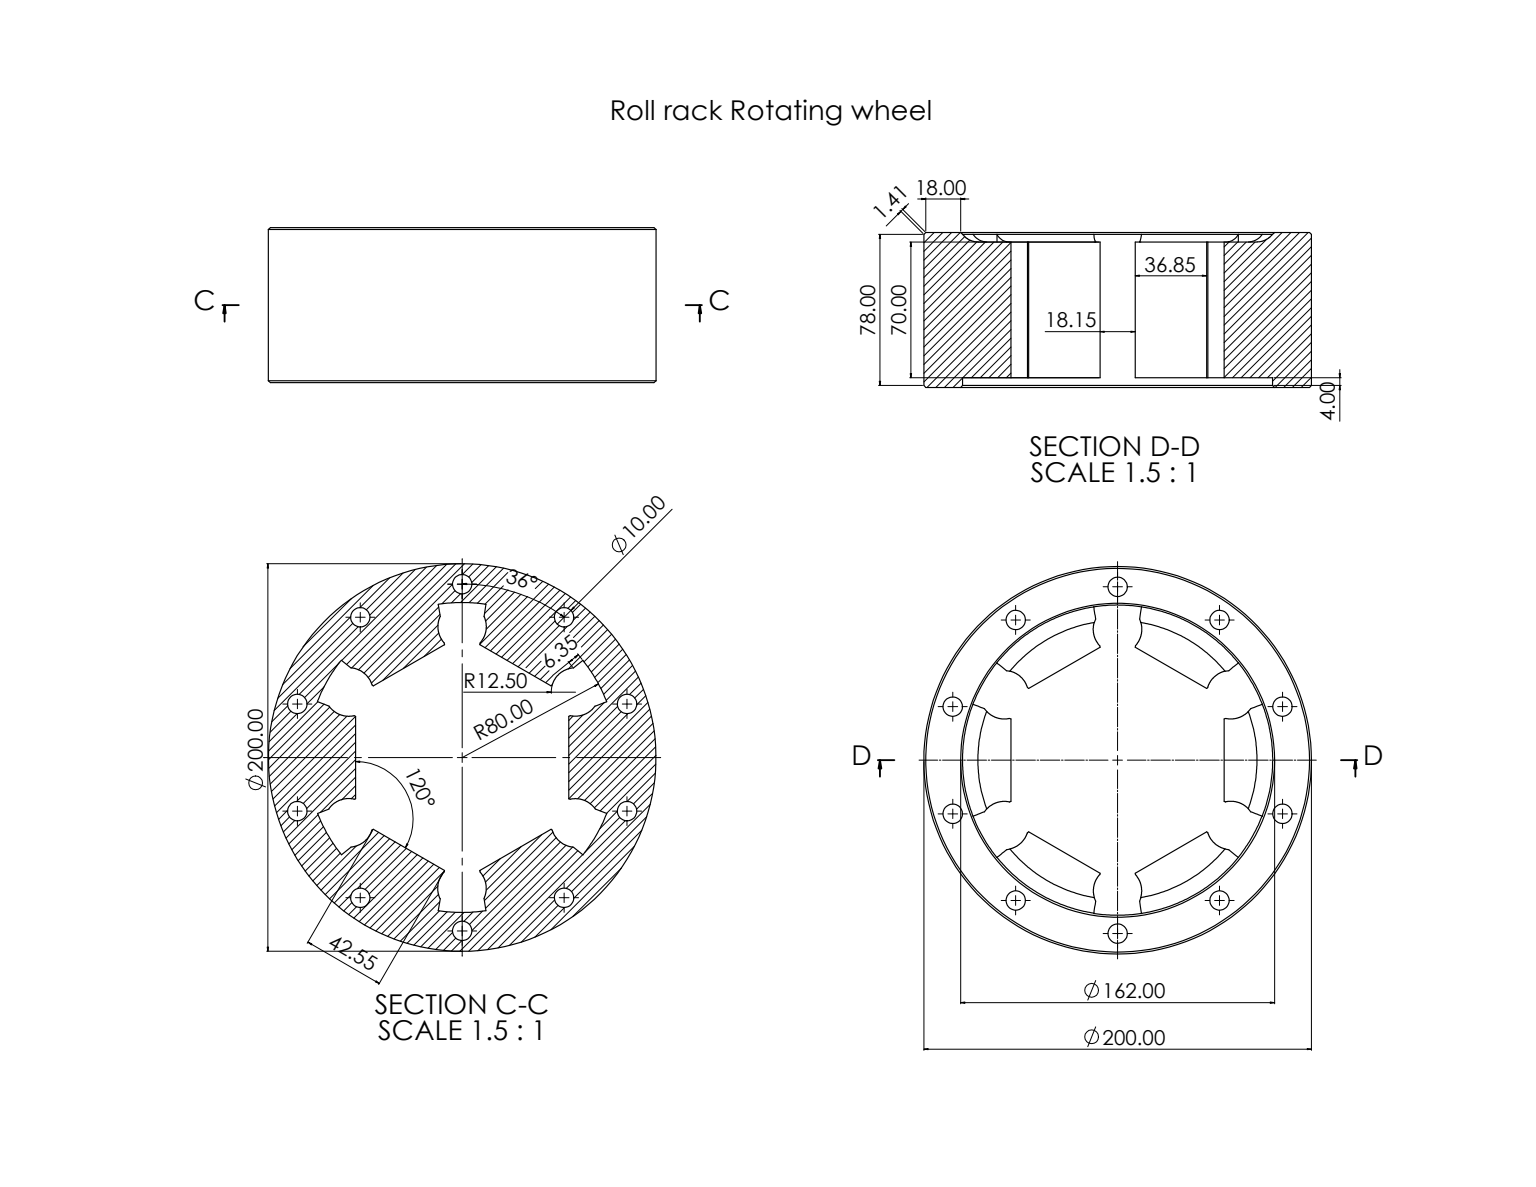
ISO-10303-21;
HEADER;
FILE_DESCRIPTION (('STEP AP214'),
    '1' );
FILE_NAME ('Roll rack Rotating wheel.step',
    '2026-10-25T19:19:31',
    ( '' ),
    ( '' ),
    'SwSTEP 2.0',
    'SolidWorks 2025',
    '' );
FILE_SCHEMA (( 'AUTOMOTIVE_DESIGN' ));
ENDSEC;

DATA;
#2=AXIS2_PLACEMENT_3D ( 'NONE', #924, #2806, #4329 ) ;
#5=ORIENTED_EDGE ( 'NONE', *, *, #469, .T. ) ;
#9=EDGE_CURVE ( 'NONE', #3175, #2261, #1933, .T. ) ;
#11=EDGE_LOOP ( 'NONE', ( #620, #96, #4571, #312 ) ) ;
#12=DIRECTION ( 'NONE',  ( 0.6273063437270283149, 0.7787725926866119197, -0.000000000000000000 ) ) ;
#15=VERTEX_POINT ( 'NONE', #3832 ) ;
#16=ORIENTED_EDGE ( 'NONE', *, *, #1748, .F. ) ;
#17=LINE ( 'NONE', #2869, #5066 ) ;
#21=EDGE_CURVE ( 'NONE', #4952, #1308, #564, .T. ) ;
#24=ORIENTED_EDGE ( 'NONE', *, *, #3439, .T. ) ;
#27=FACE_OUTER_BOUND ( 'NONE', #743, .T. ) ;
#28=ORIENTED_EDGE ( 'NONE', *, *, #3600, .T. ) ;
#29=CARTESIAN_POINT ( 'NONE',  ( -27.50000000000000355, -47.63139720814412215, 35.00000000000000000 ) ) ;
#30=CARTESIAN_POINT ( 'NONE',  ( 0.000000000000000000, -67.50000000000000000, 35.00000000000000000 ) ) ;
#32=CARTESIAN_POINT ( 'NONE',  ( -68.69027832784050247, 26.57196568621489163, 35.13717928826310555 ) ) ;
#33=ORIENTED_EDGE ( 'NONE', *, *, #1361, .F. ) ;
#34=CARTESIAN_POINT ( 'NONE',  ( 0.000000000000000000, 0.000000000000000000, -39.00000000000002842 ) ) ;
#36=DIRECTION ( 'NONE',  ( -0.000000000000000000, -0.000000000000000000, -1.000000000000000000 ) ) ;
#37=VERTEX_POINT ( 'NONE', #2442 ) ;
#42=ORIENTED_EDGE ( 'NONE', *, *, #5266, .F. ) ;
#43=ORIENTED_EDGE ( 'NONE', *, *, #3427, .F. ) ;
#44=DIRECTION ( 'NONE',  ( 1.000000000000000000, 0.000000000000000000, 0.000000000000000000 ) ) ;
#45=LINE ( 'NONE', #2928, #381 ) ;
#48=EDGE_CURVE ( 'NONE', #2705, #6084, #5252, .T. ) ;
#52=CARTESIAN_POINT ( 'NONE',  ( -85.08403291566554572, 27.64547812922971914, -40.00000000000000000 ) ) ;
#53=AXIS2_PLACEMENT_3D ( 'NONE', #2121, #1570, #3471 ) ;
#55=DIRECTION ( 'NONE',  ( -0.000000000000000000, -0.000000000000000000, -1.000000000000000000 ) ) ;
#58=AXIS2_PLACEMENT_3D ( 'NONE', #3243, #1826, #3726 ) ;
#65=AXIS2_PLACEMENT_3D ( 'NONE', #52, #3436, #1534 ) ;
#67=LINE ( 'NONE', #4284, #175 ) ;
#68=AXIS2_PLACEMENT_3D ( 'NONE', #5525, #4167, #5643 ) ;
#70=LINE ( 'NONE', #4287, #2332 ) ;
#71=ORIENTED_EDGE ( 'NONE', *, *, #3542, .T. ) ;
#72=LINE ( 'NONE', #3851, #3967 ) ;
#73=AXIS2_PLACEMENT_3D ( 'NONE', #3304, #3763, #5645 ) ;
#76=ORIENTED_EDGE ( 'NONE', *, *, #3903, .F. ) ;
#78=ORIENTED_EDGE ( 'NONE', *, *, #3494, .T. ) ;
#79=DIRECTION ( 'NONE',  ( -0.000000000000000000, -0.000000000000000000, 1.000000000000000000 ) ) ;
#84=CARTESIAN_POINT ( 'NONE',  ( 58.45671475545002949, -33.74999999999933209, 35.00000000000000000 ) ) ;
#86=VECTOR ( 'NONE', #3244, 1000.000000000000114 ) ;
#88=CARTESIAN_POINT ( 'NONE',  ( -4.130675435985315210E-14, -1.067806758184287486E-13, -35.00000000000000000 ) ) ;
#89=DIRECTION ( 'NONE',  ( -0.000000000000000000, -0.000000000000000000, 1.000000000000000000 ) ) ;
#91=ORIENTED_EDGE ( 'NONE', *, *, #553, .T. ) ;
#92=CYLINDRICAL_SURFACE ( 'NONE', #5438, 12.50000000000000355 ) ;
#93=CIRCLE ( 'NONE', #494, 100.0000000000000000 ) ;
#95=VECTOR ( 'NONE', #4136, 1000.000000000000000 ) ;
#96=ORIENTED_EDGE ( 'NONE', *, *, #2491, .F. ) ;
#97=VECTOR ( 'NONE', #2993, 1000.000000000000000 ) ;
#99=EDGE_CURVE ( 'NONE', #3250, #2370, #287, .T. ) ;
#103=VERTEX_POINT ( 'NONE', #3026 ) ;
#104=DIRECTION ( 'NONE',  ( 1.000000000000000000, 0.000000000000000000, 0.000000000000000000 ) ) ;
#106=CARTESIAN_POINT ( 'NONE',  ( 90.08403291566575888, -27.64547812922912939, -40.00000000000000000 ) ) ;
#107=ORIENTED_EDGE ( 'NONE', *, *, #3615, .T. ) ;
#110=ORIENTED_EDGE ( 'NONE', *, *, #2448, .F. ) ;
#111=ORIENTED_EDGE ( 'NONE', *, *, #3009, .T. ) ;
#112=DIRECTION ( 'NONE',  ( -1.000000000000000000, 0.000000000000000000, 0.000000000000000000 ) ) ;
#117=ORIENTED_EDGE ( 'NONE', *, *, #561, .F. ) ;
#123=ORIENTED_EDGE ( 'NONE', *, *, #596, .F. ) ;
#126=ORIENTED_EDGE ( 'NONE', *, *, #1149, .F. ) ;
#128=EDGE_CURVE ( 'NONE', #3596, #4984, #485, .T. ) ;
#130=EDGE_CURVE ( 'NONE', #3466, #5138, #2058, .T. ) ;
#132=VERTEX_POINT ( 'NONE', #187 ) ;
#135=CARTESIAN_POINT ( 'NONE',  ( 11.82353433160363387, 71.60642589802917257, 35.00000000000000000 ) ) ;
#138=EDGE_CURVE ( 'NONE', #2272, #193, #3964, .T. ) ;
#139=ORIENTED_EDGE ( 'NONE', *, *, #5184, .F. ) ;
#140=ORIENTED_EDGE ( 'NONE', *, *, #2807, .F. ) ;
#142=DIRECTION ( 'NONE',  ( -0.4999999999999919509, -0.8660254037844432595, 0.000000000000000000 ) ) ;
#143=DIRECTION ( 'NONE',  ( 0.8660254037844374864, 0.5000000000000018874, 0.000000000000000000 ) ) ;
#144=CARTESIAN_POINT ( 'NONE',  ( 55.71784976887228424, -21.55374571496028224, -35.00000000000000000 ) ) ;
#148=CARTESIAN_POINT ( 'NONE',  ( -99.00000000000005684, 0.000000000000000000, 40.00000000000000000 ) ) ;
#152=ORIENTED_EDGE ( 'NONE', *, *, #4059, .F. ) ;
#154=EDGE_CURVE ( 'NONE', #2132, #2202, #3672, .T. ) ;
#155=CIRCLE ( 'NONE', #3811, 12.50000000000138733 ) ;
#157=CARTESIAN_POINT ( 'NONE',  ( -67.92475106770436355, 25.56373185532726566, 35.00000000000000000 ) ) ;
#158=ORIENTED_EDGE ( 'NONE', *, *, #5715, .F. ) ;
#159=FACE_OUTER_BOUND ( 'NONE', #3787, .T. ) ;
#160=CIRCLE ( 'NONE', #3618, 5.000000000000004441 ) ;
#162=CIRCLE ( 'NONE', #672, 99.00000000000005684 ) ;
#163=LINE ( 'NONE', #3014, #5926 ) ;
#165=AXIS2_PLACEMENT_3D ( 'NONE', #2293, #4791, #5233 ) ;
#166=CARTESIAN_POINT ( 'NONE',  ( -90.08403291566554572, 27.64547812922971914, 40.00000000000000000 ) ) ;
#170=AXIS2_PLACEMENT_3D ( 'NONE', #2221, #6035, #3192 ) ;
#171=ORIENTED_EDGE ( 'NONE', *, *, #1511, .T. ) ;
#173=ORIENTED_EDGE ( 'NONE', *, *, #319, .F. ) ;
#174=PLANE ( 'NONE',  #2670 ) ;
#175=VECTOR ( 'NONE', #443, 1000.000000000000000 ) ;
#177=DIRECTION ( 'NONE',  ( 0.000000000000000000, 0.000000000000000000, 1.000000000000000000 ) ) ;
#179=AXIS2_PLACEMENT_3D ( 'NONE', #1316, #5314, #565 ) ;
#182=DIRECTION ( 'NONE',  ( -0.000000000000000000, -0.000000000000000000, -1.000000000000000000 ) ) ;
#183=ORIENTED_EDGE ( 'NONE', *, *, #3874, .T. ) ;
#184=VECTOR ( 'NONE', #2953, 1000.000000000000000 ) ;
#187=CARTESIAN_POINT ( 'NONE',  ( -11.33314185116896589, -72.77350886803867525, -35.00000000000000000 ) ) ;
#188=FACE_OUTER_BOUND ( 'NONE', #757, .T. ) ;
#189=AXIS2_PLACEMENT_3D ( 'NONE', #1496, #4390, #4322 ) ;
#190=ORIENTED_EDGE ( 'NONE', *, *, #4573, .T. ) ;
#191=DIRECTION ( 'NONE',  ( -1.000000000000000000, 0.000000000000000000, 0.000000000000000000 ) ) ;
#193=VERTEX_POINT ( 'NONE', #6023 ) ;
#197=AXIS2_PLACEMENT_3D ( 'NONE', #5583, #3182, #1309 ) ;
#199=EDGE_LOOP ( 'NONE', ( #4634, #1674, #4035, #780 ) ) ;
#200=CARTESIAN_POINT ( 'NONE',  ( -56.72666074499610289, 46.14586675604117971, 35.04915833130703362 ) ) ;
#201=CIRCLE ( 'NONE', #4460, 80.99999999999998579 ) ;
#204=ORIENTED_EDGE ( 'NONE', *, *, #2780, .T. ) ;
#206=ORIENTED_EDGE ( 'NONE', *, *, #6021, .F. ) ;
#208=EDGE_CURVE ( 'NONE', #3788, #4471, #2464, .T. ) ;
#209=ADVANCED_FACE ( 'NONE', ( #3211 ), #1827, .F. ) ;
#210=CARTESIAN_POINT ( 'NONE',  ( 85.08403291566575888, -27.64547812922912939, -79.99999999999998579 ) ) ;
#212=VECTOR ( 'NONE', #3452, 1000.000000000000000 ) ;
#213=LINE ( 'NONE', #3513, #2487 ) ;
#214=DIRECTION ( 'NONE',  ( -0.1538769332794359124, -0.9880900209011910240, 0.000000000000000000 ) ) ;
#216=ORIENTED_EDGE ( 'NONE', *, *, #469, .F. ) ;
#218=CARTESIAN_POINT ( 'NONE',  ( 85.08403291566575888, -27.64547812922912939, -79.99999999999998579 ) ) ;
#220=CARTESIAN_POINT ( 'NONE',  ( 58.45671475545002949, -33.74999999999933209, -35.00000000000000000 ) ) ;
#221=ORIENTED_EDGE ( 'NONE', *, *, #961, .T. ) ;
#222=CARTESIAN_POINT ( 'NONE',  ( 0.000000000000000000, 67.50000000000000000, 35.00000000000000000 ) ) ;
#227=PLANE ( 'NONE',  #262 ) ;
#228=EDGE_LOOP ( 'NONE', ( #2833, #2613, #5, #4505, #3148 ) ) ;
#229=DIRECTION ( 'NONE',  ( -0.000000000000000000, -0.000000000000000000, 1.000000000000000000 ) ) ;
#230=DIRECTION ( 'NONE',  ( 1.000000000000000000, 0.000000000000000000, 0.000000000000000000 ) ) ;
#234=ORIENTED_EDGE ( 'NONE', *, *, #392, .F. ) ;
#236=LINE ( 'NONE', #1613, #5345 ) ;
#238=CARTESIAN_POINT ( 'NONE',  ( 0.000000000000000000, 0.000000000000000000, 45.00000000000000711 ) ) ;
#239=CARTESIAN_POINT ( 'NONE',  ( -52.58482424179536707, 72.37680137756343868, 40.00000000000000000 ) ) ;
#241=EDGE_CURVE ( 'NONE', #1987, #2346, #2214, .T. ) ;
#245=PLANE ( 'NONE',  #776 ) ;
#246=ORIENTED_EDGE ( 'NONE', *, *, #2518, .T. ) ;
#247=PLANE ( 'NONE',  #2430 ) ;
#252=DIRECTION ( 'NONE',  ( -0.000000000000000000, -0.000000000000000000, -1.000000000000000000 ) ) ;
#256=ORIENTED_EDGE ( 'NONE', *, *, #1736, .F. ) ;
#257=ORIENTED_EDGE ( 'NONE', *, *, #4805, .F. ) ;
#258=VECTOR ( 'NONE', #4022, 1000.000000000000000 ) ;
#261=LINE ( 'NONE', #1193, #1745 ) ;
#262=AXIS2_PLACEMENT_3D ( 'NONE', #791, #5542, #322 ) ;
#264=CARTESIAN_POINT ( 'NONE',  ( -55.00000000000000711, -2.463307335887066074E-13, -35.00000000000000000 ) ) ;
#267=FACE_OUTER_BOUND ( 'NONE', #1954, .T. ) ;
#268=CARTESIAN_POINT ( 'NONE',  ( 58.45671475545002949, -33.74999999999933209, 35.00000000000000000 ) ) ;
#269=AXIS2_PLACEMENT_3D ( 'NONE', #1659, #727, #3101 ) ;
#270=AXIS2_PLACEMENT_3D ( 'NONE', #5191, #932, #5592 ) ;
#275=CARTESIAN_POINT ( 'NONE',  ( -57.35713647666923976, 46.20154318182412112, -35.00000000000000000 ) ) ;
#276=AXIS2_PLACEMENT_3D ( 'NONE', #3833, #3374, #536 ) ;
#277=AXIS2_PLACEMENT_3D ( 'NONE', #5004, #3496, #662 ) ;
#279=CARTESIAN_POINT ( 'NONE',  ( -99.00000000000000000, 1.218523565151616460E-14, -40.00000000000000000 ) ) ;
#282=ORIENTED_EDGE ( 'NONE', *, *, #3578, .T. ) ;
#283=AXIS2_PLACEMENT_3D ( 'NONE', #2617, #2590, #2677 ) ;
#284=PLANE ( 'NONE',  #4114 ) ;
#286=FACE_OUTER_BOUND ( 'NONE', #5823, .T. ) ;
#287=CIRCLE ( 'NONE', #788, 80.00000000000000000 ) ;
#288=FACE_OUTER_BOUND ( 'NONE', #4896, .T. ) ;
#290=ORIENTED_EDGE ( 'NONE', *, *, #3576, .F. ) ;
#291=ORIENTED_EDGE ( 'NONE', *, *, #9, .T. ) ;
#295=ORIENTED_EDGE ( 'NONE', *, *, #6012, .F. ) ;
#299=PLANE ( 'NONE',  #2579 ) ;
#300=CARTESIAN_POINT ( 'NONE',  ( 57.35713647667095927, 46.20154318182582642, 35.00000000000000000 ) ) ;
#302=AXIS2_PLACEMENT_3D ( 'NONE', #2834, #4360, #112 ) ;
#309=CIRCLE ( 'NONE', #2876, 12.49999999999999822 ) ;
#311=DIRECTION ( 'NONE',  ( -0.7787725926866080339, -0.6273063437270329779, 0.000000000000000000 ) ) ;
#312=ORIENTED_EDGE ( 'NONE', *, *, #2008, .T. ) ;
#313=PRODUCT_DEFINITION ( 'UNKNOWN', '', #4945, #1510 ) ;
#316=ORIENTED_EDGE ( 'NONE', *, *, #3343, .F. ) ;
#319=EDGE_CURVE ( 'NONE', #3286, #747, #5307, .T. ) ;
#322=DIRECTION ( 'NONE',  ( -0.9326495259660518844, 0.3607836771741465554, 0.000000000000000000 ) ) ;
#324=EDGE_CURVE ( 'NONE', #559, #1473, #4803, .T. ) ;
#326=ORIENTED_EDGE ( 'NONE', *, *, #3380, .T. ) ;
#332=LINE ( 'NONE', #833, #5327 ) ;
#334=EDGE_CURVE ( 'NONE', #2774, #836, #5704, .T. ) ;
#335=CARTESIAN_POINT ( 'NONE',  ( -45.92560378283280187, -36.99336990414421678, 35.00000000000000000 ) ) ;
#337=CARTESIAN_POINT ( 'NONE',  ( -80.00000000000000000, 9.858406733136196781E-15, 38.99999999999995737 ) ) ;
#339=DIRECTION ( 'NONE',  ( 0.8660254037844374864, 0.5000000000000018874, 0.000000000000000000 ) ) ;
#345=DIRECTION ( 'NONE',  ( 0.4999999999999979461, 0.8660254037844397068, 0.000000000000000000 ) ) ;
#346=CARTESIAN_POINT ( 'NONE',  ( 0.000000000000000000, 0.000000000000000000, -35.00000000000000000 ) ) ;
#347=CARTESIAN_POINT ( 'NONE',  ( 80.00000000000000000, 9.797174393178826052E-15, -35.00000000000000000 ) ) ;
#348=DIRECTION ( 'NONE',  ( 0.9326495259660493309, -0.3607836771741531612, 0.000000000000000000 ) ) ;
#352=ORIENTED_EDGE ( 'NONE', *, *, #5211, .T. ) ;
#355=LINE ( 'NONE', #765, #5264 ) ;
#356=LINE ( 'NONE', #854, #4752 ) ;
#357=ADVANCED_FACE ( 'NONE', ( #528 ), #1432, .F. ) ;
#358=CYLINDRICAL_SURFACE ( 'NONE', #2932, 5.000000000000005329 ) ;
#361=CIRCLE ( 'NONE', #2438, 5.000000000000003553 ) ;
#362=EDGE_LOOP ( 'NONE', ( #5160, #1425, #4288, #5479, #680 ) ) ;
#364=CYLINDRICAL_SURFACE ( 'NONE', #2030, 5.000000000000004441 ) ;
#366=EDGE_CURVE ( 'NONE', #3309, #2604, #45, .T. ) ;
#367=VECTOR ( 'NONE', #4179, 1000.000000000000000 ) ;
#371=AXIS2_PLACEMENT_3D ( 'NONE', #5124, #1347, #5615 ) ;
#372=ORIENTED_EDGE ( 'NONE', *, *, #1885, .T. ) ;
#373=AXIS2_PLACEMENT_3D ( 'NONE', #5753, #1444, #5257 ) ;
#375=DIRECTION ( 'NONE',  ( 0.1538769332794487910, -0.9880900209011889146, 0.000000000000000000 ) ) ;
#378=DIRECTION ( 'NONE',  ( 0.9880900209011890256, 0.1538769332794488465, -0.000000000000000000 ) ) ;
#379=CARTESIAN_POINT ( 'NONE',  ( -1.131281550719566266E-13, -1.761763928569765259E-14, -35.00000000000000000 ) ) ;
#381=VECTOR ( 'NONE', #2434, 1000.000000000000000 ) ;
#385=DIRECTION ( 'NONE',  ( 0.4999999999999980016, 0.8660254037844398178, 0.000000000000000000 ) ) ;
#386=DIRECTION ( 'NONE',  ( 0.7071067811865474617, 8.659560562354932858E-17, -0.7071067811865474617 ) ) ;
#387=CARTESIAN_POINT ( 'NONE',  ( 0.000000000000000000, 0.000000000000000000, -35.00000000000000000 ) ) ;
#389=CIRCLE ( 'NONE', #3743, 81.00000000000004263 ) ;
#390=CARTESIAN_POINT ( 'NONE',  ( -46.52501622030417394, 37.47620048660903080, -35.00000000000000000 ) ) ;
#391=ADVANCED_FACE ( 'NONE', ( #4837 ), #4296, .F. ) ;
#392=EDGE_CURVE ( 'NONE', #6119, #506, #4546, .T. ) ;
#393=CIRCLE ( 'NONE', #4250, 5.000000000000004441 ) ;
#394=ORIENTED_EDGE ( 'NONE', *, *, #319, .T. ) ;
#395=FACE_OUTER_BOUND ( 'NONE', #5732, .T. ) ;
#396=CARTESIAN_POINT ( 'NONE',  ( 45.92560378283280187, 36.99336990414421678, 35.00000000000000000 ) ) ;
#398=AXIS2_PLACEMENT_3D ( 'NONE', #2597, #2507, #3090 ) ;
#403=VECTOR ( 'NONE', #3278, 1000.000000000000000 ) ;
#404=VERTEX_POINT ( 'NONE', #2337 ) ;
#406=CARTESIAN_POINT ( 'NONE',  ( 57.35713647666955950, -46.20154318182373032, 35.13717928826270054 ) ) ;
#407=ORIENTED_EDGE ( 'NONE', *, *, #3155, .F. ) ;
#408=CARTESIAN_POINT ( 'NONE',  ( -47.58482424179695158, -72.37680137756228760, -79.99999999999998579 ) ) ;
#409=EDGE_CURVE ( 'NONE', #4283, #4835, #4739, .T. ) ;
#410=CARTESIAN_POINT ( 'NONE',  ( 45.92560378283317135, -36.99336990414376913, -35.00000000000000000 ) ) ;
#411=LINE ( 'NONE', #2288, #367 ) ;
#413=VERTEX_POINT ( 'NONE', #3086 ) ;
#415=EDGE_LOOP ( 'NONE', ( #3992, #873, #2536, #5412 ) ) ;
#417=CARTESIAN_POINT ( 'NONE',  ( -54.99999999999990052, -21.27605460800010206, 35.00000000000000000 ) ) ;
#418=CARTESIAN_POINT ( 'NONE',  ( 0.000000000000000000, 0.000000000000000000, 38.99999999999995737 ) ) ;
#419=ORIENTED_EDGE ( 'NONE', *, *, #6088, .T. ) ;
#421=DIRECTION ( 'NONE',  ( 0.000000000000000000, 0.000000000000000000, 1.000000000000000000 ) ) ;
#422=ORIENTED_EDGE ( 'NONE', *, *, #959, .T. ) ;
#424=DIRECTION ( 'NONE',  ( -0.000000000000000000, -0.000000000000000000, -1.000000000000000000 ) ) ;
#426=ADVANCED_FACE ( 'NONE', ( #4483 ), #2145, .F. ) ;
#428=CARTESIAN_POINT ( 'NONE',  ( 0.000000000000000000, -67.50000000000000000, 35.00000000000000000 ) ) ;
#429=VERTEX_POINT ( 'NONE', #3953 ) ;
#431=LINE ( 'NONE', #905, #1941 ) ;
#432=EDGE_CURVE ( 'NONE', #3051, #2891, #3112, .T. ) ;
#433=ADVANCED_FACE ( 'NONE', ( #2109 ), #652, .T. ) ;
#434=ORIENTED_EDGE ( 'NONE', *, *, #2926, .T. ) ;
#435=DIRECTION ( 'NONE',  ( 0.4999999999999980571, 0.8660254037844398178, 0.000000000000000000 ) ) ;
#438=EDGE_CURVE ( 'NONE', #2727, #2151, #236, .T. ) ;
#439=CARTESIAN_POINT ( 'NONE',  ( 0.000000000000000000, 0.000000000000000000, 40.00000000000000000 ) ) ;
#441=CARTESIAN_POINT ( 'NONE',  ( -9.192833548570002122, 59.02994620156853500, 35.00000000000000000 ) ) ;
#442=ORIENTED_EDGE ( 'NONE', *, *, #4598, .F. ) ;
#443=DIRECTION ( 'NONE',  ( -0.000000000000000000, -0.000000000000000000, -1.000000000000000000 ) ) ;
#446=ORIENTED_EDGE ( 'NONE', *, *, #3414, .T. ) ;
#447=DIRECTION ( 'NONE',  ( -0.9326495259660493309, 0.3607836771741531612, 0.000000000000000000 ) ) ;
#448=CARTESIAN_POINT ( 'NONE',  ( 0.000000000000000000, 0.000000000000000000, 39.00000000000007105 ) ) ;
#449=ORIENTED_EDGE ( 'NONE', *, *, #4908, .F. ) ;
#454=CARTESIAN_POINT ( 'NONE',  ( 67.15076586955507310, 25.97642475654038208, 45.00000000000000711 ) ) ;
#455=DIRECTION ( 'NONE',  ( -0.000000000000000000, -0.000000000000000000, -1.000000000000000000 ) ) ;
#456=VECTOR ( 'NONE', #3870, 1000.000000000000000 ) ;
#457=ORIENTED_EDGE ( 'NONE', *, *, #2284, .T. ) ;
#460=ORIENTED_EDGE ( 'NONE', *, *, #2064, .F. ) ;
#461=DIRECTION ( 'NONE',  ( -0.1538769332794359124, -0.9880900209011910240, 0.000000000000000000 ) ) ;
#462=CIRCLE ( 'NONE', #5923, 10.00000000000000000 ) ;
#463=CIRCLE ( 'NONE', #5827, 80.00000000000000000 ) ;
#465=CARTESIAN_POINT ( 'NONE',  ( 0.000000000000000000, 0.000000000000000000, 40.00000000000000000 ) ) ;
#469=EDGE_CURVE ( 'NONE', #4283, #4976, #5856, .T. ) ;
#470=CARTESIAN_POINT ( 'NONE',  ( 57.35713647667095927, 46.20154318182582642, -35.00000000000000000 ) ) ;
#471=AXIS2_PLACEMENT_3D ( 'NONE', #3650, #3190, #2720 ) ;
#472=CIRCLE ( 'NONE', #5133, 5.000000000000004441 ) ;
#474=CARTESIAN_POINT ( 'NONE',  ( 46.52501622030217021, 37.47620048660763103, 35.00000000000000000 ) ) ;
#477=ORIENTED_EDGE ( 'NONE', *, *, #4239, .T. ) ;
#478=DIRECTION ( 'NONE',  ( 0.000000000000000000, 0.000000000000000000, 1.000000000000000000 ) ) ;
#480=CIRCLE ( 'NONE', #3045, 5.000000000000004441 ) ;
#481=LINE ( 'NONE', #2362, #700 ) ;
#482=CYLINDRICAL_SURFACE ( 'NONE', #4115, 12.49999999999999822 ) ;
#483=ORIENTED_EDGE ( 'NONE', *, *, #1361, .T. ) ;
#484=LINE ( 'NONE', #4827, #2071 ) ;
#485=CIRCLE ( 'NONE', #982, 12.50000000000138556 ) ;
#491=DIRECTION ( 'NONE',  ( 0.7787725926866119197, -0.6273063437270283149, 0.000000000000000000 ) ) ;
#492=CARTESIAN_POINT ( 'NONE',  ( -55.71784976887420271, -21.55374571496209057, 35.00000000000000000 ) ) ;
#494=AXIS2_PLACEMENT_3D ( 'NONE', #1360, #5019, #5052 ) ;
#496=DIRECTION ( 'NONE',  ( -0.000000000000000000, -0.000000000000000000, 1.000000000000000000 ) ) ;
#501=AXIS2_PLACEMENT_3D ( 'NONE', #5606, #4101, #6017 ) ;
#503=DIRECTION ( 'NONE',  ( 4.496403249731883200E-15, -1.000000000000000000, 0.000000000000000000 ) ) ;
#504=EDGE_CURVE ( 'NONE', #1915, #1987, #3073, .T. ) ;
#505=CIRCLE ( 'NONE', #3166, 10.00000000000000178 ) ;
#506=VERTEX_POINT ( 'NONE', #1560 ) ;
#507=DIRECTION ( 'NONE',  ( -0.000000000000000000, -0.000000000000000000, -1.000000000000000000 ) ) ;
#508=CIRCLE ( 'NONE', #5964, 12.50000000000000355 ) ;
#510=CYLINDRICAL_SURFACE ( 'NONE', #4830, 12.49999999999999822 ) ;
#511=AXIS2_PLACEMENT_3D ( 'NONE', #4477, #2587, #1635 ) ;
#512=ADVANCED_FACE ( 'NONE', ( #3981 ), #3487, .F. ) ;
#517=DIRECTION ( 'NONE',  ( 0.5000000000000099920, -0.8660254037844329345, 0.000000000000000000 ) ) ;
#518=LINE ( 'NONE', #4350, #5754 ) ;
#519=FACE_OUTER_BOUND ( 'NONE', #1704, .T. ) ;
#524=ORIENTED_EDGE ( 'NONE', *, *, #5142, .T. ) ;
#528=FACE_OUTER_BOUND ( 'NONE', #1887, .T. ) ;
#530=DIRECTION ( 'NONE',  ( 0.3607836771741718129, -0.9326495259660421144, 0.000000000000000000 ) ) ;
#531=EDGE_CURVE ( 'NONE', #5256, #4984, #2504, .T. ) ;
#536=DIRECTION ( 'NONE',  ( 1.000000000000000000, 0.000000000000000000, 0.000000000000000000 ) ) ;
#537=VERTEX_POINT ( 'NONE', #4039 ) ;
#538=LINE ( 'NONE', #2882, #759 ) ;
#543=ORIENTED_EDGE ( 'NONE', *, *, #2903, .T. ) ;
#545=CARTESIAN_POINT ( 'NONE',  ( -57.58482424179695869, -72.37680137756228760, 40.00000000000000000 ) ) ;
#549=ORIENTED_EDGE ( 'NONE', *, *, #553, .F. ) ;
#552=DIRECTION ( 'NONE',  ( 1.000000000000000000, 0.000000000000000000, 0.000000000000000000 ) ) ;
#553=EDGE_CURVE ( 'NONE', #1998, #3523, #5960, .T. ) ;
#554=DIRECTION ( 'NONE',  ( 0.9326495259660492199, -0.3607836771741531612, 0.000000000000000000 ) ) ;
#557=DIRECTION ( 'NONE',  ( -1.000000000000000000, 0.000000000000000000, 0.000000000000000000 ) ) ;
#558=CARTESIAN_POINT ( 'NONE',  ( -9.192833548570215285, -59.02994620157096506, -35.00000000000000000 ) ) ;
#559=VERTEX_POINT ( 'NONE', #5493 ) ;
#560=ORIENTED_EDGE ( 'NONE', *, *, #3380, .F. ) ;
#561=EDGE_CURVE ( 'NONE', #4523, #1252, #2256, .T. ) ;
#563=B_SPLINE_CURVE_WITH_KNOTS ( 'NONE', 3,
 ( #1838, #2310, #4749, #406 ),
 .UNSPECIFIED., .F., .F.,
 ( 4, 4 ),
 ( 0.000000000000000000, 0.001907370850883698165 ),
 .UNSPECIFIED. ) ;
#564=LINE ( 'NONE', #600, #3153 ) ;
#565=DIRECTION ( 'NONE',  ( 0.5000000000000099920, -0.8660254037844328234, 0.000000000000000000 ) ) ;
#567=ORIENTED_EDGE ( 'NONE', *, *, #2161, .F. ) ;
#570=VECTOR ( 'NONE', #4474, 1000.000000000000114 ) ;
#571=CIRCLE ( 'NONE', #574, 5.000000000000004441 ) ;
#573=VECTOR ( 'NONE', #1210, 1000.000000000000000 ) ;
#574=AXIS2_PLACEMENT_3D ( 'NONE', #4413, #3909, #5042 ) ;
#577=AXIS2_PLACEMENT_3D ( 'NONE', #2190, #3584, #5527 ) ;
#578=ORIENTED_EDGE ( 'NONE', *, *, #154, .F. ) ;
#579=PLANE ( 'NONE',  #2348 ) ;
#580=CARTESIAN_POINT ( 'NONE',  ( 54.99999999999975131, 21.27605460800048576, 35.00000000000000000 ) ) ;
#581=AXIS2_PLACEMENT_3D ( 'NONE', #4822, #2458, #104 ) ;
#582=EDGE_CURVE ( 'NONE', #3886, #1816, #1139, .T. ) ;
#583=ORIENTED_EDGE ( 'NONE', *, *, #2978, .F. ) ;
#585=DIRECTION ( 'NONE',  ( 0.000000000000000000, 0.000000000000000000, 1.000000000000000000 ) ) ;
#589=CARTESIAN_POINT ( 'NONE',  ( 0.000000000000000000, 0.000000000000000000, -39.00000000000002842 ) ) ;
#590=ORIENTED_EDGE ( 'NONE', *, *, #2017, .F. ) ;
#591=FACE_OUTER_BOUND ( 'NONE', #2563, .T. ) ;
#592=CARTESIAN_POINT ( 'NONE',  ( 9.074396217167167933, 58.26942451214404173, -35.00000000000000000 ) ) ;
#593=DIRECTION ( 'NONE',  ( 1.000000000000000000, 0.000000000000000000, 0.000000000000000000 ) ) ;
#596=EDGE_CURVE ( 'NONE', #2998, #2186, #5952, .T. ) ;
#600=CARTESIAN_POINT ( 'NONE',  ( -57.58482424179535997, 72.37680137756343868, -79.99999999999998579 ) ) ;
#601=DIRECTION ( 'NONE',  ( 1.000000000000000000, 0.000000000000000000, 0.000000000000000000 ) ) ;
#602=ORIENTED_EDGE ( 'NONE', *, *, #777, .T. ) ;
#603=CARTESIAN_POINT ( 'NONE',  ( 27.50000000000000355, 47.63139720814412215, 35.00000000000000000 ) ) ;
#604=AXIS2_PLACEMENT_3D ( 'NONE', #3810, #5171, #2796 ) ;
#607=VECTOR ( 'NONE', #1106, 1000.000000000000000 ) ;
#608=ORIENTED_EDGE ( 'NONE', *, *, #1198, .T. ) ;
#611=AXIS2_PLACEMENT_3D ( 'NONE', #84, #455, #3766 ) ;
#612=ADVANCED_FACE ( 'NONE', ( #1767 ), #4186, .F. ) ;
#614=DIRECTION ( 'NONE',  ( 1.000000000000000000, 0.000000000000000000, 0.000000000000000000 ) ) ;
#616=ORIENTED_EDGE ( 'NONE', *, *, #432, .F. ) ;
#617=CARTESIAN_POINT ( 'NONE',  ( -56.10121673609948090, 46.04269404270066701, 35.00000000000000000 ) ) ;
#620=ORIENTED_EDGE ( 'NONE', *, *, #2697, .F. ) ;
#622=ORIENTED_EDGE ( 'NONE', *, *, #582, .T. ) ;
#623=CARTESIAN_POINT ( 'NONE',  ( -74.61196207728391983, 28.86269417393235415, -35.00000000000000000 ) ) ;
#625=FACE_OUTER_BOUND ( 'NONE', #3417, .T. ) ;
#626=DIRECTION ( 'NONE',  ( 0.000000000000000000, 0.000000000000000000, 1.000000000000000000 ) ) ;
#629=DIRECTION ( 'NONE',  ( 0.5000000000000103251, -0.8660254037844326014, 0.000000000000000000 ) ) ;
#630=ORIENTED_EDGE ( 'NONE', *, *, #2851, .T. ) ;
#631=ORIENTED_EDGE ( 'NONE', *, *, #1846, .F. ) ;
#634=CARTESIAN_POINT ( 'NONE',  ( -56.72666074499684896, -46.14586675604289212, 35.04915833130718994 ) ) ;
#635=EDGE_CURVE ( 'NONE', #3286, #4672, #1728, .T. ) ;
#637=FACE_OUTER_BOUND ( 'NONE', #3669, .T. ) ;
#639=ORIENTED_EDGE ( 'NONE', *, *, #959, .F. ) ;
#641=EDGE_CURVE ( 'NONE', #3470, #836, #1329, .T. ) ;
#644=ORIENTED_EDGE ( 'NONE', *, *, #1662, .F. ) ;
#645=CARTESIAN_POINT ( 'NONE',  ( -1.630640067418198669E-13, 67.50000000000002842, 35.00000000000000000 ) ) ;
#648=ORIENTED_EDGE ( 'NONE', *, *, #4917, .T. ) ;
#651=DIRECTION ( 'NONE',  ( -0.000000000000000000, -0.000000000000000000, 1.000000000000000000 ) ) ;
#652=PLANE ( 'NONE',  #5646 ) ;
#655=CYLINDRICAL_SURFACE ( 'NONE', #3963, 5.000000000000004441 ) ;
#656=VERTEX_POINT ( 'NONE', #417 ) ;
#658=LINE ( 'NONE', #396, #3915 ) ;
#659=DIRECTION ( 'NONE',  ( 1.000000000000000000, 0.000000000000000000, 0.000000000000000000 ) ) ;
#660=DIRECTION ( 'NONE',  ( -0.5000000000000019984, 0.8660254037844375974, 0.000000000000000000 ) ) ;
#661=EDGE_LOOP ( 'NONE', ( #1061, #4979, #2915, #140, #3754, #1581, #2888, #2462, #2821, #639, #1009, #3061, #3078, #887, #3758, #1992 ) ) ;
#662=DIRECTION ( 'NONE',  ( 0.1538769332794358846, 0.9880900209011910240, 0.000000000000000000 ) ) ;
#666=CIRCLE ( 'NONE', #1719, 5.000000000000004441 ) ;
#670=VERTEX_POINT ( 'NONE', #3233 ) ;
#672=AXIS2_PLACEMENT_3D ( 'NONE', #3089, #1561, #4041 ) ;
#674=CARTESIAN_POINT ( 'NONE',  ( 0.000000000000000000, 0.000000000000000000, 40.00000000000000000 ) ) ;
#677=CIRCLE ( 'NONE', #4732, 5.000000000000005329 ) ;
#679=CARTESIAN_POINT ( 'NONE',  ( 62.30180741492871022, 50.18450749816254586, 38.99999999999995737 ) ) ;
#680=ORIENTED_EDGE ( 'NONE', *, *, #2232, .T. ) ;
#681=CARTESIAN_POINT ( 'NONE',  ( 54.99999999999975131, 21.27605460800048576, -35.00000000000000000 ) ) ;
#682=CIRCLE ( 'NONE', #778, 4.999999999999990230 ) ;
#683=DIRECTION ( 'NONE',  ( 0.3607836771741718684, -0.9326495259660421144, 0.000000000000000000 ) ) ;
#685=FACE_OUTER_BOUND ( 'NONE', #2877, .T. ) ;
#691=( NAMED_UNIT ( * ) PLANE_ANGLE_UNIT ( ) SI_UNIT ( $, .RADIAN. ) );
#693=DIRECTION ( 'NONE',  ( 1.154631945610162802E-14, -1.000000000000000000, 0.000000000000000000 ) ) ;
#697=CARTESIAN_POINT ( 'NONE',  ( 57.58482424179591419, -72.37680137756305498, -79.99999999999998579 ) ) ;
#698=EDGE_CURVE ( 'NONE', #2060, #2569, #1468, .T. ) ;
#699=DIRECTION ( 'NONE',  ( 0.9326495259660493309, -0.3607836771741531612, 0.000000000000000000 ) ) ;
#700=VECTOR ( 'NONE', #2496, 1000.000000000000000 ) ;
#701=B_SPLINE_CURVE_WITH_KNOTS ( 'NONE', 3,
 ( #3878, #4820, #3382, #5294 ),
 .UNSPECIFIED., .F., .F.,
 ( 4, 4 ),
 ( 0.000000000000000000, 0.001907370850886569132 ),
 .UNSPECIFIED. ) ;
#703=CIRCLE ( 'NONE', #1276, 5.000000000000004441 ) ;
#704=DIRECTION ( 'NONE',  ( 1.000000000000000000, 0.000000000000000000, 0.000000000000000000 ) ) ;
#705=VERTEX_POINT ( 'NONE', #4161 ) ;
#708=EDGE_CURVE ( 'NONE', #2370, #5794, #356, .T. ) ;
#709=DIRECTION ( 'NONE',  ( -0.8660254037844339337, -0.5000000000000079936, 0.000000000000000000 ) ) ;
#710=AXIS2_PLACEMENT_3D ( 'NONE', #1909, #3290, #2419 ) ;
#713=ORIENTED_EDGE ( 'NONE', *, *, #1737, .T. ) ;
#715=DIRECTION ( 'NONE',  ( 0.000000000000000000, 0.000000000000000000, 1.000000000000000000 ) ) ;
#719=VERTEX_POINT ( 'NONE', #6045 ) ;
#722=CARTESIAN_POINT ( 'NONE',  ( 0.000000000000000000, 0.000000000000000000, -39.00000000000001421 ) ) ;
#723=EDGE_CURVE ( 'NONE', #2393, #4821, #2733, .T. ) ;
#724=ORIENTED_EDGE ( 'NONE', *, *, #4597, .T. ) ;
#727=DIRECTION ( 'NONE',  ( 0.000000000000000000, 0.000000000000000000, 1.000000000000000000 ) ) ;
#730=VERTEX_POINT ( 'NONE', #6073 ) ;
#732=CARTESIAN_POINT ( 'NONE',  ( 99.00000000000000000, 0.000000000000000000, -40.00000000000000000 ) ) ;
#734=ORIENTED_EDGE ( 'NONE', *, *, #4098, .T. ) ;
#736=EDGE_LOOP ( 'NONE', ( #1054, #1574, #5921, #216, #1999, #3686, #5636 ) ) ;
#738=CARTESIAN_POINT ( 'NONE',  ( -58.45671475544979501, 33.74999999999974420, 35.00000000000000000 ) ) ;
#740=CARTESIAN_POINT ( 'NONE',  ( -57.35713647666923976, 46.20154318182412112, 35.13717928826270054 ) ) ;
#741=CARTESIAN_POINT ( 'NONE',  ( -58.45671475544946816, -33.75000000000027711, -35.00000000000000000 ) ) ;
#742=EDGE_CURVE ( 'NONE', #5503, #2020, #5457, .T. ) ;
#743=EDGE_LOOP ( 'NONE', ( #123, #3043, #1631, #4334 ) ) ;
#747=VERTEX_POINT ( 'NONE', #5634 ) ;
#748=CARTESIAN_POINT ( 'NONE',  ( -62.30180741492891627, 50.18450749816232559, -35.00000000000000711 ) ) ;
#749=EDGE_CURVE ( 'NONE', #2774, #3309, #93, .T. ) ;
#753=FACE_BOUND ( 'NONE', #1300, .T. ) ;
#756=ORIENTED_EDGE ( 'NONE', *, *, #2983, .F. ) ;
#757=EDGE_LOOP ( 'NONE', ( #1083, #1609, #1805, #974, #3958 ) ) ;
#759=VECTOR ( 'NONE', #5814, 1000.000000000000114 ) ;
#762=DIRECTION ( 'NONE',  ( 1.000000000000000000, 0.000000000000000000, 0.000000000000000000 ) ) ;
#765=CARTESIAN_POINT ( 'NONE',  ( 7.182140071210238271E-14, -8.916303653273167033E-14, -35.00000000000000000 ) ) ;
#769=DIRECTION ( 'NONE',  ( 0.000000000000000000, 0.000000000000000000, 1.000000000000000000 ) ) ;
#771=ORIENTED_EDGE ( 'NONE', *, *, #5079, .T. ) ;
#775=DIRECTION ( 'NONE',  ( -0.7787725926866081450, -0.6273063437270328668, 0.000000000000000000 ) ) ;
#776=AXIS2_PLACEMENT_3D ( 'NONE', #4465, #4518, #311 ) ;
#777=EDGE_CURVE ( 'NONE', #5916, #5503, #4544, .T. ) ;
#778=AXIS2_PLACEMENT_3D ( 'NONE', #3943, #2076, #5392 ) ;
#780=ORIENTED_EDGE ( 'NONE', *, *, #3835, .F. ) ;
#784=ORIENTED_EDGE ( 'NONE', *, *, #438, .F. ) ;
#786=CARTESIAN_POINT ( 'NONE',  ( 0.000000000000000000, 0.000000000000000000, -39.00000000000002842 ) ) ;
#787=EDGE_CURVE ( 'NONE', #2393, #1473, #5668, .T. ) ;
#788=AXIS2_PLACEMENT_3D ( 'NONE', #722, #4046, #659 ) ;
#790=AXIS2_PLACEMENT_3D ( 'NONE', #1923, #3303, #593 ) ;
#791=CARTESIAN_POINT ( 'NONE',  ( -4.130675435985315210E-14, -1.067806758184287486E-13, 35.00000000000000000 ) ) ;
#792=ORIENTED_EDGE ( 'NONE', *, *, #641, .F. ) ;
#794=AXIS2_PLACEMENT_3D ( 'NONE', #2565, #4454, #4637 ) ;
#796=ORIENTED_EDGE ( 'NONE', *, *, #3047, .T. ) ;
#797=CARTESIAN_POINT ( 'NONE',  ( 67.92475106770271509, 25.56373185532915926, 35.00000000000000000 ) ) ;
#798=CIRCLE ( 'NONE', #5654, 4.999999999999997335 ) ;
#799=ORIENTED_EDGE ( 'NONE', *, *, #787, .F. ) ;
#800=DIRECTION ( 'NONE',  ( 1.000000000000000000, 0.000000000000000000, 0.000000000000000000 ) ) ;
#802=CIRCLE ( 'NONE', #3651, 5.000000000000004441 ) ;
#804=DIRECTION ( 'NONE',  ( -0.7787725926866118087, 0.6273063437270282039, 0.000000000000000000 ) ) ;
#807=DIRECTION ( 'NONE',  ( -0.7787725926866080339, -0.6273063437270329779, 0.000000000000000000 ) ) ;
#808=ORIENTED_EDGE ( 'NONE', *, *, #6021, .T. ) ;
#816=VERTEX_POINT ( 'NONE', #3780 ) ;
#818=EDGE_CURVE ( 'NONE', #4790, #2604, #4823, .T. ) ;
#819=DIRECTION ( 'NONE',  ( -0.7071067811865474617, 8.659560562354932858E-17, 0.7071067811865474617 ) ) ;
#823=DIRECTION ( 'NONE',  ( -0.7787725926866162496, 0.6273063437270229858, 0.000000000000000000 ) ) ;
#824=EDGE_LOOP ( 'NONE', ( #1358, #407, #4198, #2211 ) ) ;
#828=ORIENTED_EDGE ( 'NONE', *, *, #4445, .T. ) ;
#830=ORIENTED_EDGE ( 'NONE', *, *, #3407, .F. ) ;
#831=DIRECTION ( 'NONE',  ( -0.000000000000000000, 0.000000000000000000, 1.000000000000000000 ) ) ;
#832=DIRECTION ( 'NONE',  ( -0.000000000000000000, -0.000000000000000000, -1.000000000000000000 ) ) ;
#833=CARTESIAN_POINT ( 'NONE',  ( 27.50000000000043698, -47.63139720814386635, 35.00000000000000000 ) ) ;
#836=VERTEX_POINT ( 'NONE', #2889 ) ;
#837=CARTESIAN_POINT ( 'NONE',  ( 0.000000000000000000, 0.000000000000000000, 38.99999999999995737 ) ) ;
#838=DIRECTION ( 'NONE',  ( -0.000000000000000000, -0.000000000000000000, -1.000000000000000000 ) ) ;
#842=ORIENTED_EDGE ( 'NONE', *, *, #5142, .F. ) ;
#844=CARTESIAN_POINT ( 'NONE',  ( 47.58482424179590708, -72.37680137756305498, 40.00000000000000000 ) ) ;
#845=CARTESIAN_POINT ( 'NONE',  ( 74.61196207728340823, 28.86269417393367220, -35.00000000000000711 ) ) ;
#848=EDGE_CURVE ( 'NONE', #3788, #2202, #518, .T. ) ;
#850=CARTESIAN_POINT ( 'NONE',  ( 62.30180741492923602, -50.18450749816189216, 35.00000000000000000 ) ) ;
#851=ORIENTED_EDGE ( 'NONE', *, *, #3535, .F. ) ;
#852=LINE ( 'NONE', #911, #5350 ) ;
#854=CARTESIAN_POINT ( 'NONE',  ( 80.99999999999998579, 9.919639073093559622E-15, -40.00000000000000000 ) ) ;
#855=DIRECTION ( 'NONE',  ( 1.000000000000000000, 0.000000000000000000, 0.000000000000000000 ) ) ;
#858=DIRECTION ( 'NONE',  ( -0.000000000000000000, -0.000000000000000000, -1.000000000000000000 ) ) ;
#860=AXIS2_PLACEMENT_3D ( 'NONE', #418, #2296, #5237 ) ;
#861=ORIENTED_EDGE ( 'NONE', *, *, #2673, .F. ) ;
#862=DIRECTION ( 'NONE',  ( 1.000000000000000000, 0.000000000000000000, 0.000000000000000000 ) ) ;
#868=CIRCLE ( 'NONE', #4025, 80.00000000000000000 ) ;
#869=ORIENTED_EDGE ( 'NONE', *, *, #1198, .F. ) ;
#872=CARTESIAN_POINT ( 'NONE',  ( -81.00000000000004263, 9.919639073093567511E-15, 40.00000000000000000 ) ) ;
#873=ORIENTED_EDGE ( 'NONE', *, *, #708, .T. ) ;
#876=CIRCLE ( 'NONE', #5445, 5.000000000000004441 ) ;
#877=DIRECTION ( 'NONE',  ( 1.000000000000000000, 0.000000000000000000, 0.000000000000000000 ) ) ;
#878=DIRECTION ( 'NONE',  ( -1.000000000000000000, 0.000000000000000000, 0.000000000000000000 ) ) ;
#880=EDGE_LOOP ( 'NONE', ( #2654, #2905, #5186, #326 ) ) ;
#881=CARTESIAN_POINT ( 'NONE',  ( -4.130675435985315210E-14, -1.067806758184287486E-13, 35.00000000000000000 ) ) ;
#883=CARTESIAN_POINT ( 'NONE',  ( 85.08403291566575888, -27.64547812922912939, -40.00000000000000000 ) ) ;
#887=ORIENTED_EDGE ( 'NONE', *, *, #2926, .F. ) ;
#889=AXIS2_PLACEMENT_3D ( 'NONE', #5137, #3747, #4633 ) ;
#890=DIRECTION ( 'NONE',  ( 0.000000000000000000, 0.000000000000000000, -1.000000000000000000 ) ) ;
#892=ORIENTED_EDGE ( 'NONE', *, *, #3835, .T. ) ;
#894=DIRECTION ( 'NONE',  ( -0.000000000000000000, -0.000000000000000000, -1.000000000000000000 ) ) ;
#899=VECTOR ( 'NONE', #4486, 1000.000000000000000 ) ;
#902=ORIENTED_EDGE ( 'NONE', *, *, #6125, .T. ) ;
#905=CARTESIAN_POINT ( 'NONE',  ( 8.056095891487838412E-14, -1.254589464284425060E-14, 35.00000000000000000 ) ) ;
#906=VERTEX_POINT ( 'NONE', #545 ) ;
#911=CARTESIAN_POINT ( 'NONE',  ( 74.61196207728410457, -28.86269417393182479, 35.00000000000000000 ) ) ;
#912=ORIENTED_EDGE ( 'NONE', *, *, #6122, .F. ) ;
#913=DIRECTION ( 'NONE',  ( 1.000000000000000000, 1.154631945610162960E-14, -0.000000000000000000 ) ) ;
#914=DIRECTION ( 'NONE',  ( -0.6273063437270228748, -0.7787725926866162496, 0.000000000000000000 ) ) ;
#916=DIRECTION ( 'NONE',  ( -0.7787725926866118087, 0.6273063437270282039, 0.000000000000000000 ) ) ;
#917=DIRECTION ( 'NONE',  ( -0.000000000000000000, -0.000000000000000000, -1.000000000000000000 ) ) ;
#918=ORIENTED_EDGE ( 'NONE', *, *, #1893, .T. ) ;
#919=ORIENTED_EDGE ( 'NONE', *, *, #5150, .F. ) ;
#921=CARTESIAN_POINT ( 'NONE',  ( -57.58482424179535997, 72.37680137756343868, -40.00000000000000000 ) ) ;
#924=CARTESIAN_POINT ( 'NONE',  ( 0.000000000000000000, 0.000000000000000000, 45.00000000000000711 ) ) ;
#926=ADVANCED_FACE ( 'NONE', ( #940 ), #2825, .F. ) ;
#931=ORIENTED_EDGE ( 'NONE', *, *, #2696, .F. ) ;
#932=DIRECTION ( 'NONE',  ( -0.000000000000000000, 0.000000000000000000, 1.000000000000000000 ) ) ;
#933=ADVANCED_FACE ( 'NONE', ( #5767 ), #1912, .T. ) ;
#934=DIRECTION ( 'NONE',  ( 0.000000000000000000, -1.000000000000000000, 0.000000000000000000 ) ) ;
#935=CARTESIAN_POINT ( 'NONE',  ( -90.08403291566611415, -27.64547812922793923, -79.99999999999998579 ) ) ;
#937=LINE ( 'NONE', #1390, #2653 ) ;
#938=ORIENTED_EDGE ( 'NONE', *, *, #3903, .T. ) ;
#940=FACE_OUTER_BOUND ( 'NONE', #2415, .T. ) ;
#941=DIRECTION ( 'NONE',  ( -0.7787725926866080339, -0.6273063437270329779, 0.000000000000000000 ) ) ;
#946=EDGE_CURVE ( 'NONE', #656, #5782, #1457, .T. ) ;
#947=EDGE_LOOP ( 'NONE', ( #1531, #1314, #3935, #3872, #5576 ) ) ;
#948=LINE ( 'NONE', #2335, #4654 ) ;
#953=DIRECTION ( 'NONE',  ( 0.6273063437270329779, -0.7787725926866080339, 0.000000000000000000 ) ) ;
#954=AXIS2_PLACEMENT_3D ( 'NONE', #2303, #2213, #1775 ) ;
#959=EDGE_CURVE ( 'NONE', #5881, #2218, #481, .T. ) ;
#960=VECTOR ( 'NONE', #1277, 1000.000000000000227 ) ;
#961=EDGE_CURVE ( 'NONE', #3596, #5854, #2473, .T. ) ;
#963=CARTESIAN_POINT ( 'NONE',  ( -55.48030965892933608, -45.89047003626479437, 35.00000000000000000 ) ) ;
#965=AXIS2_PLACEMENT_3D ( 'NONE', #2285, #3254, #4203 ) ;
#967=DIRECTION ( 'NONE',  ( 1.000000000000000000, 0.000000000000000000, 0.000000000000000000 ) ) ;
#969=AXIS2_PLACEMENT_3D ( 'NONE', #3897, #4783, #3342 ) ;
#971=CARTESIAN_POINT ( 'NONE',  ( 0.000000000000000000, 89.46264649666795776, -40.00000000000000000 ) ) ;
#974=ORIENTED_EDGE ( 'NONE', *, *, #504, .T. ) ;
#975=CARTESIAN_POINT ( 'NONE',  ( 67.48246767247886169, -25.10212255632678691, 35.00000000000000000 ) ) ;
#976=VECTOR ( 'NONE', #3280, 999.9999999999998863 ) ;
#977=ADVANCED_FACE ( 'NONE', ( #2013 ), #4384, .F. ) ;
#979=CARTESIAN_POINT ( 'NONE',  ( 58.45671475544962448, 33.75000000000001421, 35.00000000000000000 ) ) ;
#980=ORIENTED_EDGE ( 'NONE', *, *, #1593, .T. ) ;
#981=DIRECTION ( 'NONE',  ( -0.000000000000000000, -0.000000000000000000, -1.000000000000000000 ) ) ;
#982=AXIS2_PLACEMENT_3D ( 'NONE', #2154, #3583, #5500 ) ;
#985=ORIENTED_EDGE ( 'NONE', *, *, #3040, .T. ) ;
#987=CARTESIAN_POINT ( 'NONE',  ( 4.130675435985391572E-14, 1.067806758184284836E-13, -35.00000000000000000 ) ) ;
#989=VECTOR ( 'NONE', #3356, 1000.000000000000000 ) ;
#990=FACE_OUTER_BOUND ( 'NONE', #5026, .T. ) ;
#993=VERTEX_POINT ( 'NONE', #1338 ) ;
#998=ORIENTED_EDGE ( 'NONE', *, *, #5906, .F. ) ;
#1000=B_SPLINE_CURVE_WITH_KNOTS ( 'NONE', 3,
 ( #5349, #634, #3868, #1440 ),
 .UNSPECIFIED., .F., .F.,
 ( 4, 4 ),
 ( 0.000000000000000000, 0.001907370850886569132 ),
 .UNSPECIFIED. ) ;
#1004=TOROIDAL_SURFACE ( 'NONE', #3270, 72.00000000000004263, 10.00000000000000000 ) ;
#1006=EDGE_CURVE ( 'NONE', #5881, #6071, #4043, .T. ) ;
#1007=LINE ( 'NONE', #474, #4657 ) ;
#1009=ORIENTED_EDGE ( 'NONE', *, *, #1006, .T. ) ;
#1010=DIRECTION ( 'NONE',  ( 1.000000000000000000, 0.000000000000000000, 0.000000000000000000 ) ) ;
#1013=VERTEX_POINT ( 'NONE', #3118 ) ;
#1015=ADVANCED_FACE ( 'NONE', ( #5059 ), #6079, .F. ) ;
#1018=DIRECTION ( 'NONE',  ( -1.000000000000000000, 0.000000000000000000, 0.000000000000000000 ) ) ;
#1021=CARTESIAN_POINT ( 'NONE',  ( -47.58482424179536707, 72.37680137756343868, -79.99999999999998579 ) ) ;
#1029=DIRECTION ( 'NONE',  ( 0.000000000000000000, -0.000000000000000000, -1.000000000000000000 ) ) ;
#1030=ORIENTED_EDGE ( 'NONE', *, *, #4531, .T. ) ;
#1031=DIRECTION ( 'NONE',  ( -0.000000000000000000, -0.000000000000000000, -1.000000000000000000 ) ) ;
#1039=EDGE_CURVE ( 'NONE', #5910, #413, #4673, .T. ) ;
#1041=CARTESIAN_POINT ( 'NONE',  ( 57.58482424179591419, -72.37680137756305498, -40.00000000000000000 ) ) ;
#1043=FACE_BOUND ( 'NONE', #1489, .T. ) ;
#1045=EDGE_LOOP ( 'NONE', ( #1790, #4583, #2088, #3942, #117, #3049 ) ) ;
#1046=VERTEX_POINT ( 'NONE', #4140 ) ;
#1047=FACE_OUTER_BOUND ( 'NONE', #5958, .T. ) ;
#1048=CARTESIAN_POINT ( 'NONE',  ( 56.07162667343639839, -45.16605674834566742, 45.00000000000000711 ) ) ;
#1052=CARTESIAN_POINT ( 'NONE',  ( 55.48030965892933608, 45.89047003626479437, 35.00000000000000000 ) ) ;
#1054=ORIENTED_EDGE ( 'NONE', *, *, #504, .F. ) ;
#1058=CYLINDRICAL_SURFACE ( 'NONE', #6124, 5.000000000000004441 ) ;
#1059=ADVANCED_FACE ( 'NONE', ( #395 ), #2240, .F. ) ;
#1061=ORIENTED_EDGE ( 'NONE', *, *, #5883, .T. ) ;
#1062=DIRECTION ( 'NONE',  ( -1.000000000000000000, 0.000000000000000000, 0.000000000000000000 ) ) ;
#1064=AXIS2_PLACEMENT_3D ( 'NONE', #3822, #1156, #1865 ) ;
#1065=ORIENTED_EDGE ( 'NONE', *, *, #5850, .F. ) ;
#1066=CIRCLE ( 'NONE', #860, 80.00000000000000000 ) ;
#1068=AXIS2_PLACEMENT_3D ( 'NONE', #2222, #6038, #3656 ) ;
#1069=CIRCLE ( 'NONE', #2550, 80.00000000000000000 ) ;
#1073=ORIENTED_EDGE ( 'NONE', *, *, #2636, .T. ) ;
#1074=CARTESIAN_POINT ( 'NONE',  ( 57.58482424179643999, 72.37680137756268550, -79.99999999999998579 ) ) ;
#1076=( NAMED_UNIT ( * ) SI_UNIT ( $, .STERADIAN. ) SOLID_ANGLE_UNIT ( ) );
#1077=VERTEX_POINT ( 'NONE', #3725 ) ;
#1080=AXIS2_PLACEMENT_3D ( 'NONE', #2782, #2961, #1018 ) ;
#1082=ORIENTED_EDGE ( 'NONE', *, *, #1930, .F. ) ;
#1083=ORIENTED_EDGE ( 'NONE', *, *, #4408, .F. ) ;
#1085=DIRECTION ( 'NONE',  ( -0.3607836771741652626, 0.9326495259660446679, 0.000000000000000000 ) ) ;
#1090=AXIS2_PLACEMENT_3D ( 'NONE', #2994, #715, #5927 ) ;
#1091=EDGE_LOOP ( 'NONE', ( #4998, #5006, #372, #5083 ) ) ;
#1093=DIRECTION ( 'NONE',  ( -0.000000000000000000, -0.000000000000000000, 1.000000000000000000 ) ) ;
#1095=EDGE_LOOP ( 'NONE', ( #5196, #583, #892, #2898 ) ) ;
#1096=DIRECTION ( 'NONE',  ( -0.000000000000000000, 0.000000000000000000, 1.000000000000000000 ) ) ;
#1097=VECTOR ( 'NONE', #832, 1000.000000000000000 ) ;
#1100=VECTOR ( 'NONE', #2822, 999.9999999999998863 ) ;
#1101=ORIENTED_EDGE ( 'NONE', *, *, #5455, .T. ) ;
#1102=VECTOR ( 'NONE', #5245, 1000.000000000000000 ) ;
#1104=CIRCLE ( 'NONE', #710, 9.999999999999992895 ) ;
#1106=DIRECTION ( 'NONE',  ( 0.7071067811865524577, 8.659560562354994488E-17, -0.7071067811865426878 ) ) ;
#1109=CARTESIAN_POINT ( 'NONE',  ( -55.00000000000010658, 21.27605460799956205, -35.00000000000000000 ) ) ;
#1112=ORIENTED_EDGE ( 'NONE', *, *, #48, .F. ) ;
#1113=ORIENTED_EDGE ( 'NONE', *, *, #2696, .T. ) ;
#1115=DIRECTION ( 'NONE',  ( 1.000000000000000000, 0.000000000000000000, 0.000000000000000000 ) ) ;
#1118=EDGE_LOOP ( 'NONE', ( #158, #442, #3485, #918 ) ) ;
#1121=DIRECTION ( 'NONE',  ( -0.8660254037844374864, -0.5000000000000018874, 0.000000000000000000 ) ) ;
#1124=EDGE_LOOP ( 'NONE', ( #3007, #2372, #4915, #1849 ) ) ;
#1125=CARTESIAN_POINT ( 'NONE',  ( 0.000000000000000000, 0.000000000000000000, 45.00000000000000711 ) ) ;
#1129=EDGE_CURVE ( 'NONE', #5138, #4037, #1779, .T. ) ;
#1132=DIRECTION ( 'NONE',  ( 0.8660254037844385966, -0.5000000000000001110, 0.000000000000000000 ) ) ;
#1133=DIRECTION ( 'NONE',  ( 1.000000000000000000, 0.000000000000000000, 0.000000000000000000 ) ) ;
#1135=VERTEX_POINT ( 'NONE', #337 ) ;
#1139=LINE ( 'NONE', #3020, #3162 ) ;
#1141=CYLINDRICAL_SURFACE ( 'NONE', #1376, 5.000000000000005329 ) ;
#1142=DIRECTION ( 'NONE',  ( 0.000000000000000000, 0.000000000000000000, 1.000000000000000000 ) ) ;
#1146=EDGE_LOOP ( 'NONE', ( #4649, #2011, #4947, #457, #71 ) ) ;
#1149=EDGE_CURVE ( 'NONE', #2239, #2101, #505, .T. ) ;
#1151=FACE_OUTER_BOUND ( 'NONE', #4461, .T. ) ;
#1153=AXIS2_PLACEMENT_3D ( 'NONE', #5021, #769, #2651 ) ;
#1155=EDGE_CURVE ( 'NONE', #4960, #3906, #3068, .T. ) ;
#1156=DIRECTION ( 'NONE',  ( 0.000000000000000000, 0.000000000000000000, 1.000000000000000000 ) ) ;
#1158=LINE ( 'NONE', #2987, #1257 ) ;
#1161=AXIS2_PLACEMENT_3D ( 'NONE', #3524, #3586, #191 ) ;
#1163=ORIENTED_EDGE ( 'NONE', *, *, #3170, .F. ) ;
#1164=DIRECTION ( 'NONE',  ( -1.000000000000000000, 0.000000000000000000, 0.000000000000000000 ) ) ;
#1165=VERTEX_POINT ( 'NONE', #5776 ) ;
#1169=CARTESIAN_POINT ( 'NONE',  ( -27.50000000000010303, 47.63139720814406530, -35.00000000000000000 ) ) ;
#1170=CYLINDRICAL_SURFACE ( 'NONE', #1867, 5.000000000000004441 ) ;
#1172=ORIENTED_EDGE ( 'NONE', *, *, #582, .F. ) ;
#1175=ORIENTED_EDGE ( 'NONE', *, *, #5364, .T. ) ;
#1176=DIRECTION ( 'NONE',  ( -0.000000000000000000, -0.000000000000000000, -1.000000000000000000 ) ) ;
#1179=DIRECTION ( 'NONE',  ( -0.000000000000000000, -0.000000000000000000, -1.000000000000000000 ) ) ;
#1180=AXIS2_PLACEMENT_3D ( 'NONE', #837, #5115, #862 ) ;
#1183=AXIS2_PLACEMENT_3D ( 'NONE', #4482, #4422, #2054 ) ;
#1185=VERTEX_POINT ( 'NONE', #3365 ) ;
#1187=AXIS2_PLACEMENT_3D ( 'NONE', #4904, #683, #5898 ) ;
#1188=EDGE_CURVE ( 'NONE', #404, #1798, #2373, .T. ) ;
#1193=CARTESIAN_POINT ( 'NONE',  ( -46.52501622030217021, -37.47620048660763103, 35.00000000000000000 ) ) ;
#1195=DIRECTION ( 'NONE',  ( -0.000000000000000000, 0.000000000000000000, 1.000000000000000000 ) ) ;
#1198=EDGE_CURVE ( 'NONE', #4858, #2502, #2371, .T. ) ;
#1199=DIRECTION ( 'NONE',  ( 1.000000000000000000, 0.000000000000000000, 0.000000000000000000 ) ) ;
#1200=EDGE_CURVE ( 'NONE', #4821, #705, #948, .T. ) ;
#1201=LINE ( 'NONE', #4042, #899 ) ;
#1202=VERTEX_POINT ( 'NONE', #3330 ) ;
#1207=CARTESIAN_POINT ( 'NONE',  ( 99.00000000000005684, 1.218523565151616775E-14, 40.00000000000000000 ) ) ;
#1210=DIRECTION ( 'NONE',  ( -0.000000000000000000, -0.000000000000000000, 1.000000000000000000 ) ) ;
#1217=ORIENTED_EDGE ( 'NONE', *, *, #432, .T. ) ;
#1218=CARTESIAN_POINT ( 'NONE',  ( -11.33314185116958051, 72.77350886804100583, 35.00000000000000000 ) ) ;
#1219=ORIENTED_EDGE ( 'NONE', *, *, #5913, .T. ) ;
#1220=DIRECTION ( 'NONE',  ( -0.000000000000000000, -0.000000000000000000, -1.000000000000000000 ) ) ;
#1223=CARTESIAN_POINT ( 'NONE',  ( 0.000000000000000000, 0.000000000000000000, 35.00000000000000000 ) ) ;
#1224=CARTESIAN_POINT ( 'NONE',  ( 5.000000000000003553, 89.46264649666795776, -40.00000000000000000 ) ) ;
#1226=ORIENTED_EDGE ( 'NONE', *, *, #3873, .T. ) ;
#1228=EDGE_CURVE ( 'NONE', #1202, #2489, #17, .T. ) ;
#1232=ORIENTED_EDGE ( 'NONE', *, *, #5079, .F. ) ;
#1234=ORIENTED_EDGE ( 'NONE', *, *, #3885, .T. ) ;
#1235=ADVANCED_FACE ( 'NONE', ( #1047 ), #4774, .T. ) ;
#1238=CARTESIAN_POINT ( 'NONE',  ( 12.31015466235579225, -79.04720167209512738, -35.00000000000000000 ) ) ;
#1244=DIRECTION ( 'NONE',  ( 0.5000000000000101030, -0.8660254037844328234, 0.000000000000000000 ) ) ;
#1246=DIRECTION ( 'NONE',  ( 0.7071067811865573427, 0.000000000000000000, 0.7071067811865378028 ) ) ;
#1250=CIRCLE ( 'NONE', #269, 80.00000000000000000 ) ;
#1251=ADVANCED_FACE ( 'NONE', ( #2404 ), #1402, .F. ) ;
#1252=VERTEX_POINT ( 'NONE', #2925 ) ;
#1256=CARTESIAN_POINT ( 'NONE',  ( 12.31015466235579581, -79.04720167209514159, 38.99999999999995737 ) ) ;
#1257=VECTOR ( 'NONE', #229, 1000.000000000000000 ) ;
#1260=EDGE_CURVE ( 'NONE', #4988, #4357, #802, .T. ) ;
#1264=FACE_BOUND ( 'NONE', #2991, .T. ) ;
#1266=EDGE_CURVE ( 'NONE', #1046, #4044, #5961, .T. ) ;
#1267=PLANE ( 'NONE',  #4208 ) ;
#1269=AXIS2_PLACEMENT_3D ( 'NONE', #3631, #4666, #385 ) ;
#1271=EDGE_LOOP ( 'NONE', ( #3181, #5939 ) ) ;
#1273=EDGE_LOOP ( 'NONE', ( #543, #808 ) ) ;
#1274=LINE ( 'NONE', #5018, #5757 ) ;
#1276=AXIS2_PLACEMENT_3D ( 'NONE', #5398, #3888, #2107 ) ;
#1277=DIRECTION ( 'NONE',  ( 0.1538769332794487910, -0.9880900209011889146, 0.000000000000000000 ) ) ;
#1279=AXIS2_PLACEMENT_3D ( 'NONE', #239, #4513, #5930 ) ;
#1280=DIRECTION ( 'NONE',  ( -0.000000000000000000, -0.000000000000000000, -1.000000000000000000 ) ) ;
#1281=ORIENTED_EDGE ( 'NONE', *, *, #5948, .T. ) ;
#1288=VERTEX_POINT ( 'NONE', #3789 ) ;
#1290=DIRECTION ( 'NONE',  ( -1.000000000000000000, -4.496403249731883200E-15, 0.000000000000000000 ) ) ;
#1291=ADVANCED_FACE ( 'NONE', ( #2432 ), #3394, .T. ) ;
#1292=ADVANCED_FACE ( 'NONE', ( #591 ), #2469, .F. ) ;
#1293=CARTESIAN_POINT ( 'NONE',  ( 0.000000000000000000, 0.000000000000000000, 38.99999999999995737 ) ) ;
#1296=FACE_OUTER_BOUND ( 'NONE', #11, .T. ) ;
#1299=LINE ( 'NONE', #850, #1763 ) ;
#1300=EDGE_LOOP ( 'NONE', ( #5701, #608 ) ) ;
#1303=FACE_OUTER_BOUND ( 'NONE', #3931, .T. ) ;
#1305=DIRECTION ( 'NONE',  ( -0.8660254037844385966, 0.5000000000000001110, 0.000000000000000000 ) ) ;
#1307=PLANE ( 'NONE',  #3165 ) ;
#1308=VERTEX_POINT ( 'NONE', #3084 ) ;
#1309=DIRECTION ( 'NONE',  ( 0.4999999999999976685, 0.8660254037844400399, 0.000000000000000000 ) ) ;
#1310=CARTESIAN_POINT ( 'NONE',  ( 57.58482424179643999, 72.37680137756268550, 40.00000000000000000 ) ) ;
#1314=ORIENTED_EDGE ( 'NONE', *, *, #3282, .T. ) ;
#1316=CARTESIAN_POINT ( 'NONE',  ( 0.000000000000000000, 0.000000000000000000, -35.00000000000000000 ) ) ;
#1317=CARTESIAN_POINT ( 'NONE',  ( -58.45671475544979501, 33.74999999999974420, -35.00000000000000000 ) ) ;
#1318=EDGE_CURVE ( 'NONE', #5782, #1798, #5425, .T. ) ;
#1319=DIRECTION ( 'NONE',  ( -0.1538769332794488187, 0.9880900209011889146, 0.000000000000000000 ) ) ;
#1320=DIRECTION ( 'NONE',  ( 0.000000000000000000, 0.000000000000000000, -1.000000000000000000 ) ) ;
#1322=EDGE_CURVE ( 'NONE', #4090, #3660, #703, .T. ) ;
#1323=EDGE_CURVE ( 'NONE', #4821, #1077, #1612, .T. ) ;
#1327=ORIENTED_EDGE ( 'NONE', *, *, #130, .T. ) ;
#1329=LINE ( 'NONE', #5578, #1854 ) ;
#1330=AXIS2_PLACEMENT_3D ( 'NONE', #3347, #1096, #1479 ) ;
#1331=FACE_OUTER_BOUND ( 'NONE', #880, .T. ) ;
#1333=EDGE_CURVE ( 'NONE', #4672, #2051, #2503, .T. ) ;
#1334=LINE ( 'NONE', #1735, #95 ) ;
#1336=VECTOR ( 'NONE', #3920, 1000.000000000000000 ) ;
#1337=EDGE_LOOP ( 'NONE', ( #1724, #6116, #4750, #792 ) ) ;
#1338=CARTESIAN_POINT ( 'NONE',  ( 47.58482424179590708, -72.37680137756305498, -40.00000000000000000 ) ) ;
#1341=CIRCLE ( 'NONE', #2444, 80.00000000000000000 ) ;
#1344=AXIS2_PLACEMENT_3D ( 'NONE', #1708, #3556, #2603 ) ;
#1347=DIRECTION ( 'NONE',  ( -0.000000000000000000, -0.000000000000000000, -1.000000000000000000 ) ) ;
#1353=DIRECTION ( 'NONE',  ( -0.000000000000000000, -0.000000000000000000, -1.000000000000000000 ) ) ;
#1356=AXIS2_PLACEMENT_3D ( 'NONE', #2406, #1085, #3791 ) ;
#1357=PLANE ( 'NONE',  #1843 ) ;
#1358=ORIENTED_EDGE ( 'NONE', *, *, #1857, .T. ) ;
#1359=FACE_OUTER_BOUND ( 'NONE', #1337, .T. ) ;
#1360=CARTESIAN_POINT ( 'NONE',  ( 0.000000000000000000, 0.000000000000000000, 39.00000000000007105 ) ) ;
#1361=EDGE_CURVE ( 'NONE', #4312, #3660, #2619, .T. ) ;
#1363=ORIENTED_EDGE ( 'NONE', *, *, #1913, .T. ) ;
#1365=CONICAL_SURFACE ( 'NONE', #3654, 99.00000000000005684, 0.7853981633974552734 ) ;
#1367=AXIS2_PLACEMENT_3D ( 'NONE', #1699, #5987, #6010 ) ;
#1368=VERTEX_POINT ( 'NONE', #4961 ) ;
#1369=DIRECTION ( 'NONE',  ( 1.000000000000000000, 0.000000000000000000, 0.000000000000000000 ) ) ;
#1370=DIRECTION ( 'NONE',  ( 0.000000000000000000, 0.000000000000000000, 1.000000000000000000 ) ) ;
#1373=EDGE_CURVE ( 'NONE', #4037, #1523, #4758, .T. ) ;
#1374=CARTESIAN_POINT ( 'NONE',  ( -45.92560378283280187, -36.99336990414421678, 35.00000000000000000 ) ) ;
#1376=AXIS2_PLACEMENT_3D ( 'NONE', #2596, #4395, #1199 ) ;
#1377=ORIENTED_EDGE ( 'NONE', *, *, #4999, .T. ) ;
#1379=ORIENTED_EDGE ( 'NONE', *, *, #2734, .T. ) ;
#1380=DIRECTION ( 'NONE',  ( -0.6273063437270228748, -0.7787725926866162496, 0.000000000000000000 ) ) ;
#1381=ORIENTED_EDGE ( 'NONE', *, *, #3194, .T. ) ;
#1382=CARTESIAN_POINT ( 'NONE',  ( 68.69027832783777399, 26.57196568621521138, 35.13717928826270054 ) ) ;
#1384=CARTESIAN_POINT ( 'NONE',  ( -62.30180741492871022, -50.18450749816254586, 35.00000000000000000 ) ) ;
#1385=UNCERTAINTY_MEASURE_WITH_UNIT (LENGTH_MEASURE( 1.000000000000000082E-05 ), #5406, 'distance_accuracy_value', 'NONE');
#1389=EDGE_LOOP ( 'NONE', ( #5861, #91, #4233, #4006 ) ) ;
#1390=CARTESIAN_POINT ( 'NONE',  ( 1.131281550719567528E-13, 1.761763928569687004E-14, 35.00000000000000000 ) ) ;
#1391=EDGE_LOOP ( 'NONE', ( #76, #1113, #4616, #460 ) ) ;
#1394=CYLINDRICAL_SURFACE ( 'NONE', #4719, 5.000000000000003553 ) ;
#1397=CARTESIAN_POINT ( 'NONE',  ( 100.0000000000000000, 1.224646799147353217E-14, 39.00000000000007105 ) ) ;
#1400=ORIENTED_EDGE ( 'NONE', *, *, #1748, .T. ) ;
#1402=CYLINDRICAL_SURFACE ( 'NONE', #2971, 5.000000000000004441 ) ;
#1403=CARTESIAN_POINT ( 'NONE',  ( -11.33314185116958051, 72.77350886804100583, 35.13717928826310555 ) ) ;
#1406=CARTESIAN_POINT ( 'NONE',  ( -74.61196207728360719, -28.86269417393314995, 35.00000000000000000 ) ) ;
#1409=EDGE_LOOP ( 'NONE', ( #5433, #2142, #3328, #3543 ) ) ;
#1412=FACE_OUTER_BOUND ( 'NONE', #3433, .T. ) ;
#1415=EDGE_CURVE ( 'NONE', #1915, #3734, #1664, .T. ) ;
#1422=CARTESIAN_POINT ( 'NONE',  ( 45.92560378283280187, 36.99336990414421678, -35.00000000000000000 ) ) ;
#1425=ORIENTED_EDGE ( 'NONE', *, *, #2852, .F. ) ;
#1428=ORIENTED_EDGE ( 'NONE', *, *, #561, .T. ) ;
#1429=EDGE_LOOP ( 'NONE', ( #234, #3916, #5684, #1556 ) ) ;
#1430=DIRECTION ( 'NONE',  ( -0.000000000000000000, -0.000000000000000000, -1.000000000000000000 ) ) ;
#1432=PLANE ( 'NONE',  #1356 ) ;
#1434=ADVANCED_FACE ( 'NONE', ( #3546 ), #174, .F. ) ;
#1435=FACE_OUTER_BOUND ( 'NONE', #1990, .T. ) ;
#1436=AXIS2_PLACEMENT_3D ( 'NONE', #1048, #5416, #5246 ) ;
#1437=ORIENTED_EDGE ( 'NONE', *, *, #531, .T. ) ;
#1440=CARTESIAN_POINT ( 'NONE',  ( -55.48030965892933608, -45.89047003626479437, 35.00000000000000000 ) ) ;
#1441=MECHANICAL_DESIGN_GEOMETRIC_PRESENTATION_REPRESENTATION('',(#2545),#5126);
#1442=EDGE_CURVE ( 'NONE', #3100, #2065, #4052, .T. ) ;
#1443=ORIENTED_EDGE ( 'NONE', *, *, #2208, .F. ) ;
#1444=DIRECTION ( 'NONE',  ( 0.9880900209011910240, -0.1538769332794358846, 0.000000000000000000 ) ) ;
#1445=CIRCLE ( 'NONE', #4942, 80.00000000000000000 ) ;
#1447=CIRCLE ( 'NONE', #581, 80.00000000000000000 ) ;
#1448=DIRECTION ( 'NONE',  ( 1.000000000000000000, 0.000000000000000000, 0.000000000000000000 ) ) ;
#1450=EDGE_CURVE ( 'NONE', #1368, #5498, #1759, .T. ) ;
#1455=ORIENTED_EDGE ( 'NONE', *, *, #366, .T. ) ;
#1456=CARTESIAN_POINT ( 'NONE',  ( 68.69027832784067300, -26.57196568621440491, 35.13717928826310555 ) ) ;
#1457=LINE ( 'NONE', #2916, #3060 ) ;
#1458=FACE_OUTER_BOUND ( 'NONE', #2159, .T. ) ;
#1460=DIRECTION ( 'NONE',  ( -0.4999999999999920619, -0.8660254037844431485, 0.000000000000000000 ) ) ;
#1462=ORIENTED_EDGE ( 'NONE', *, *, #749, .F. ) ;
#1464=DIRECTION ( 'NONE',  ( -0.000000000000000000, 0.000000000000000000, 1.000000000000000000 ) ) ;
#1468=CIRCLE ( 'NONE', #1660, 12.49999999999999822 ) ;
#1469=FACE_OUTER_BOUND ( 'NONE', #1389, .T. ) ;
#1471=AXIS2_PLACEMENT_3D ( 'NONE', #1791, #5197, #4601 ) ;
#1473=VERTEX_POINT ( 'NONE', #681 ) ;
#1475=VECTOR ( 'NONE', #917, 1000.000000000000000 ) ;
#1478=ORIENTED_EDGE ( 'NONE', *, *, #4270, .F. ) ;
#1479=DIRECTION ( 'NONE',  ( 1.000000000000000000, 0.000000000000000000, 0.000000000000000000 ) ) ;
#1482=ADVANCED_FACE ( 'NONE', ( #625 ), #2648, .F. ) ;
#1483=EDGE_CURVE ( 'NONE', #4960, #2705, #1274, .T. ) ;
#1486=DIRECTION ( 'NONE',  ( -0.000000000000000000, -0.000000000000000000, -1.000000000000000000 ) ) ;
#1487=EDGE_CURVE ( 'NONE', #4312, #1918, #393, .T. ) ;
#1489=EDGE_LOOP ( 'NONE', ( #5089, #5421 ) ) ;
#1491=EDGE_LOOP ( 'NONE', ( #4814, #190 ) ) ;
#1492=FACE_BOUND ( 'NONE', #2170, .T. ) ;
#1495=VERTEX_POINT ( 'NONE', #4070 ) ;
#1496=CARTESIAN_POINT ( 'NONE',  ( -1.630640067418198669E-13, 67.50000000000002842, -35.00000000000000000 ) ) ;
#1497=ORIENTED_EDGE ( 'NONE', *, *, #208, .T. ) ;
#1498=CARTESIAN_POINT ( 'NONE',  ( -55.00000000000010658, 21.27605460799956205, 35.00000000000000000 ) ) ;
#1501=DIRECTION ( 'NONE',  ( 1.000000000000000000, 0.000000000000000000, 0.000000000000000000 ) ) ;
#1503=ORIENTED_EDGE ( 'NONE', *, *, #1519, .F. ) ;
#1506=DIRECTION ( 'NONE',  ( 0.000000000000000000, 0.000000000000000000, 1.000000000000000000 ) ) ;
#1507=ORIENTED_EDGE ( 'NONE', *, *, #1228, .F. ) ;
#1508=CARTESIAN_POINT ( 'NONE',  ( -52.58482424179536707, 72.37680137756343868, -40.00000000000000000 ) ) ;
#1510=PRODUCT_DEFINITION_CONTEXT ( 'detailed design', #4404, 'design' ) ;
#1511=EDGE_CURVE ( 'NONE', #1523, #2445, #3848, .T. ) ;
#1513=FACE_OUTER_BOUND ( 'NONE', #4493, .T. ) ;
#1514=ORIENTED_EDGE ( 'NONE', *, *, #4495, .F. ) ;
#1515=LINE ( 'NONE', #2044, #2144 ) ;
#1516=DIRECTION ( 'NONE',  ( -0.000000000000000000, 0.000000000000000000, 1.000000000000000000 ) ) ;
#1517=CARTESIAN_POINT ( 'NONE',  ( 0.000000000000000000, 89.46264649666795776, 40.00000000000000000 ) ) ;
#1518=ORIENTED_EDGE ( 'NONE', *, *, #946, .F. ) ;
#1519=EDGE_CURVE ( 'NONE', #3265, #3338, #3744, .T. ) ;
#1523=VERTEX_POINT ( 'NONE', #2766 ) ;
#1528=ADVANCED_FACE ( 'NONE', ( #2679 ), #2706, .T. ) ;
#1531=ORIENTED_EDGE ( 'NONE', *, *, #1373, .T. ) ;
#1534=DIRECTION ( 'NONE',  ( 1.000000000000000000, 0.000000000000000000, 0.000000000000000000 ) ) ;
#1535=AXIS2_PLACEMENT_3D ( 'NONE', #218, #2089, #5028 ) ;
#1536=ORIENTED_EDGE ( 'NONE', *, *, #3030, .T. ) ;
#1539=VECTOR ( 'NONE', #3565, 1000.000000000000000 ) ;
#1543=TOROIDAL_SURFACE ( 'NONE', #5037, 72.00000000000004263, 10.00000000000000000 ) ;
#1546=DIRECTION ( 'NONE',  ( 0.7787725926866081450, 0.6273063437270328668, 0.000000000000000000 ) ) ;
#1547=CIRCLE ( 'NONE', #3933, 99.00000000000000000 ) ;
#1548=VERTEX_POINT ( 'NONE', #2265 ) ;
#1549=DIRECTION ( 'NONE',  ( 0.9326495259660518844, -0.3607836771741464998, 0.000000000000000000 ) ) ;
#1551=DIRECTION ( 'NONE',  ( 0.000000000000000000, 0.000000000000000000, 1.000000000000000000 ) ) ;
#1556=ORIENTED_EDGE ( 'NONE', *, *, #4137, .F. ) ;
#1557=DIRECTION ( 'NONE',  ( 0.000000000000000000, 0.000000000000000000, 1.000000000000000000 ) ) ;
#1558=EDGE_CURVE ( 'NONE', #6127, #4523, #4469, .T. ) ;
#1559=ADVANCED_FACE ( 'NONE', ( #1303 ), #3663, .F. ) ;
#1560=CARTESIAN_POINT ( 'NONE',  ( 4.999999999999380940, -89.46264649666795776, -40.00000000000000000 ) ) ;
#1561=DIRECTION ( 'NONE',  ( -0.000000000000000000, 0.000000000000000000, 1.000000000000000000 ) ) ;
#1562=CARTESIAN_POINT ( 'NONE',  ( 1.131281550719567528E-13, 1.761763928569687004E-14, -35.00000000000000000 ) ) ;
#1563=VECTOR ( 'NONE', #5339, 1000.000000000000227 ) ;
#1564=ORIENTED_EDGE ( 'NONE', *, *, #409, .T. ) ;
#1566=DIRECTION ( 'NONE',  ( 0.000000000000000000, 0.000000000000000000, 1.000000000000000000 ) ) ;
#1570=DIRECTION ( 'NONE',  ( -0.000000000000000000, -0.000000000000000000, 1.000000000000000000 ) ) ;
#1573=CIRCLE ( 'NONE', #5462, 80.00000000000000000 ) ;
#1574=ORIENTED_EDGE ( 'NONE', *, *, #1415, .T. ) ;
#1577=VECTOR ( 'NONE', #214, 999.9999999999998863 ) ;
#1581=ORIENTED_EDGE ( 'NONE', *, *, #3578, .F. ) ;
#1582=CYLINDRICAL_SURFACE ( 'NONE', #5938, 12.50000000000139089 ) ;
#1585=EDGE_LOOP ( 'NONE', ( #5295, #2692, #771, #3509 ) ) ;
#1586=DIRECTION ( 'NONE',  ( -0.000000000000000000, -0.000000000000000000, -1.000000000000000000 ) ) ;
#1587=EDGE_LOOP ( 'NONE', ( #2607, #2798, #246, #206 ) ) ;
#1589=DIRECTION ( 'NONE',  ( -0.5000000000000037748, 0.8660254037844365982, 0.000000000000000000 ) ) ;
#1590=CARTESIAN_POINT ( 'NONE',  ( 7.182140071210238271E-14, -8.916303653273167033E-14, -35.00000000000000000 ) ) ;
#1592=EDGE_CURVE ( 'NONE', #3297, #2393, #4603, .T. ) ;
#1593=EDGE_CURVE ( 'NONE', #5503, #719, #355, .T. ) ;
#1598=CARTESIAN_POINT ( 'NONE',  ( 54.99999999999999289, 6.349087922075113966E-13, -35.00000000000000000 ) ) ;
#1599=ADVANCED_FACE ( 'NONE', ( #3231 ), #299, .T. ) ;
#1602=PLANE ( 'NONE',  #5833 ) ;
#1603=EDGE_CURVE ( 'NONE', #1883, #2239, #4416, .T. ) ;
#1607=DIRECTION ( 'NONE',  ( -0.5000000000000001110, -0.8660254037844385966, 0.000000000000000000 ) ) ;
#1609=ORIENTED_EDGE ( 'NONE', *, *, #1039, .F. ) ;
#1610=CARTESIAN_POINT ( 'NONE',  ( 68.69027832783777399, 26.57196568621521138, 35.13717928826270054 ) ) ;
#1612=LINE ( 'NONE', #5837, #97 ) ;
#1613=CARTESIAN_POINT ( 'NONE',  ( -74.61196207728391983, 28.86269417393235415, 35.00000000000000000 ) ) ;
#1615=CARTESIAN_POINT ( 'NONE',  ( -68.69027832783800136, -26.57196568621473531, 35.13717928826270054 ) ) ;
#1616=CARTESIAN_POINT ( 'NONE',  ( 55.71784976887228424, -21.55374571496028224, 35.00000000000000000 ) ) ;
#1617=ORIENTED_EDGE ( 'NONE', *, *, #5715, .T. ) ;
#1623=EDGE_LOOP ( 'NONE', ( #3718, #5012, #796, #422 ) ) ;
#1624=LINE ( 'NONE', #1689, #3327 ) ;
#1625=EDGE_CURVE ( 'NONE', #3297, #15, #5041, .T. ) ;
#1626=CIRCLE ( 'NONE', #1064, 80.00000000000000000 ) ;
#1630=CARTESIAN_POINT ( 'NONE',  ( 85.08403291566575888, -27.64547812922912939, 40.00000000000000000 ) ) ;
#1631=ORIENTED_EDGE ( 'NONE', *, *, #1930, .T. ) ;
#1634=AXIS2_PLACEMENT_3D ( 'NONE', #4660, #5720, #1448 ) ;
#1635=DIRECTION ( 'NONE',  ( 0.1538769332794359679, 0.9880900209011910240, 0.000000000000000000 ) ) ;
#1637=CIRCLE ( 'NONE', #276, 100.0000000000000000 ) ;
#1638=ORIENTED_EDGE ( 'NONE', *, *, #3009, .F. ) ;
#1640=ORIENTED_EDGE ( 'NONE', *, *, #4260, .T. ) ;
#1645=CARTESIAN_POINT ( 'NONE',  ( 62.30180741492871022, 50.18450749816254586, 35.00000000000000000 ) ) ;
#1646=DIRECTION ( 'NONE',  ( -0.000000000000000000, -0.000000000000000000, 1.000000000000000000 ) ) ;
#1647=ORIENTED_EDGE ( 'NONE', *, *, #1592, .F. ) ;
#1648=TOROIDAL_SURFACE ( 'NONE', #1080, 72.00000000000004263, 10.00000000000000000 ) ;
#1650=CARTESIAN_POINT ( 'NONE',  ( 47.58482424179642578, 72.37680137756268550, -40.00000000000000000 ) ) ;
#1652=CARTESIAN_POINT ( 'NONE',  ( -58.45671475544979501, 33.74999999999974420, 35.00000000000000000 ) ) ;
#1655=DIRECTION ( 'NONE',  ( -0.3607836771741652626, 0.9326495259660446679, 0.000000000000000000 ) ) ;
#1658=ORIENTED_EDGE ( 'NONE', *, *, #5791, .T. ) ;
#1659=CARTESIAN_POINT ( 'NONE',  ( 0.000000000000000000, 0.000000000000000000, 38.99999999999995737 ) ) ;
#1660=AXIS2_PLACEMENT_3D ( 'NONE', #3177, #3716, #2680 ) ;
#1661=AXIS2_PLACEMENT_3D ( 'NONE', #4698, #3299, #5581 ) ;
#1662=EDGE_CURVE ( 'NONE', #4523, #816, #3531, .T. ) ;
#1663=EDGE_CURVE ( 'NONE', #993, #5773, #1951, .T. ) ;
#1664=CIRCLE ( 'NONE', #1183, 72.00000000000004263 ) ;
#1666=ORIENTED_EDGE ( 'NONE', *, *, #2629, .F. ) ;
#1668=AXIS2_PLACEMENT_3D ( 'NONE', #4807, #953, #2875 ) ;
#1669=EDGE_CURVE ( 'NONE', #5346, #4900, #67, .T. ) ;
#1674=ORIENTED_EDGE ( 'NONE', *, *, #5649, .T. ) ;
#1676=CARTESIAN_POINT ( 'NONE',  ( 12.31015466235495026, 79.04720167209526949, 35.00000000000000000 ) ) ;
#1678=CARTESIAN_POINT ( 'NONE',  ( 62.30180741492925733, -50.18450749816190637, -35.00000000000000711 ) ) ;
#1679=DIRECTION ( 'NONE',  ( -0.5000000000000042188, 0.8660254037844362651, 0.000000000000000000 ) ) ;
#1681=VERTEX_POINT ( 'NONE', #5199 ) ;
#1684=DIRECTION ( 'NONE',  ( 0.000000000000000000, 0.000000000000000000, 1.000000000000000000 ) ) ;
#1685=ORIENTED_EDGE ( 'NONE', *, *, #3910, .T. ) ;
#1688=EDGE_LOOP ( 'NONE', ( #3440, #2097, #3588, #3386 ) ) ;
#1689=CARTESIAN_POINT ( 'NONE',  ( -57.58482424179695869, -72.37680137756228760, -79.99999999999998579 ) ) ;
#1690=CARTESIAN_POINT ( 'NONE',  ( 11.60016251788559849, 72.19966265504864111, 35.04915833130703362 ) ) ;
#1694=EDGE_CURVE ( 'NONE', #2123, #3856, #3625, .T. ) ;
#1699=CARTESIAN_POINT ( 'NONE',  ( 27.50000000000043698, -47.63139720814386635, 35.00000000000000000 ) ) ;
#1701=ADVANCED_FACE ( 'NONE', ( #4693 ), #2824, .F. ) ;
#1702=DIRECTION ( 'NONE',  ( 0.000000000000000000, 0.000000000000000000, 1.000000000000000000 ) ) ;
#1703=DIRECTION ( 'NONE',  ( 0.000000000000000000, 0.000000000000000000, 1.000000000000000000 ) ) ;
#1704=EDGE_LOOP ( 'NONE', ( #4055, #1172, #2244, #434 ) ) ;
#1705=CARTESIAN_POINT ( 'NONE',  ( -11.33314185116958051, 72.77350886804100583, 35.13717928826310555 ) ) ;
#1708=CARTESIAN_POINT ( 'NONE',  ( 0.000000000000000000, 0.000000000000000000, -40.00000000000000000 ) ) ;
#1709=ADVANCED_FACE ( 'NONE', ( #6098 ), #5632, .F. ) ;
#1713=VERTEX_POINT ( 'NONE', #1422 ) ;
#1714=FACE_OUTER_BOUND ( 'NONE', #661, .T. ) ;
#1716=CARTESIAN_POINT ( 'NONE',  ( -1.131281550719566266E-13, -1.761763928569765259E-14, 35.00000000000000000 ) ) ;
#1719=AXIS2_PLACEMENT_3D ( 'NONE', #1630, #2639, #5452 ) ;
#1721=ORIENTED_EDGE ( 'NONE', *, *, #2318, .T. ) ;
#1722=DIRECTION ( 'NONE',  ( 1.000000000000000000, 0.000000000000000000, 0.000000000000000000 ) ) ;
#1723=VECTOR ( 'NONE', #252, 1000.000000000000000 ) ;
#1724=ORIENTED_EDGE ( 'NONE', *, *, #4091, .F. ) ;
#1726=DIRECTION ( 'NONE',  ( 0.000000000000000000, 0.000000000000000000, 1.000000000000000000 ) ) ;
#1728=LINE ( 'NONE', #3664, #1097 ) ;
#1730=AXIS2_PLACEMENT_3D ( 'NONE', #4764, #3779, #1817 ) ;
#1733=CIRCLE ( 'NONE', #1833, 99.00000000000005684 ) ;
#1734=AXIS2_PLACEMENT_3D ( 'NONE', #1317, #585, #3705 ) ;
#1735=CARTESIAN_POINT ( 'NONE',  ( -57.35713647667095927, -46.20154318182582642, 35.00000000000000000 ) ) ;
#1736=EDGE_CURVE ( 'NONE', #3734, #4976, #3621, .T. ) ;
#1737=EDGE_CURVE ( 'NONE', #4211, #3523, #3332, .T. ) ;
#1738=ORIENTED_EDGE ( 'NONE', *, *, #4727, .F. ) ;
#1742=DIRECTION ( 'NONE',  ( -0.9326495259660447790, -0.3607836771741651516, 0.000000000000000000 ) ) ;
#1743=VECTOR ( 'NONE', #651, 1000.000000000000000 ) ;
#1745=VECTOR ( 'NONE', #1586, 1000.000000000000000 ) ;
#1748=EDGE_CURVE ( 'NONE', #2101, #5574, #4607, .T. ) ;
#1750=ORIENTED_EDGE ( 'NONE', *, *, #3047, .F. ) ;
#1751=AXIS2_PLACEMENT_3D ( 'NONE', #428, #4197, #1164 ) ;
#1753=CARTESIAN_POINT ( 'NONE',  ( -11.82353433160363387, -71.60642589802917257, 35.00000000000000000 ) ) ;
#1754=LINE ( 'NONE', #5568, #3336 ) ;
#1756=DIRECTION ( 'NONE',  ( 1.000000000000000000, 0.000000000000000000, 0.000000000000000000 ) ) ;
#1757=VECTOR ( 'NONE', #2460, 1000.000000000000000 ) ;
#1759=CIRCLE ( 'NONE', #3464, 4.999999999999990230 ) ;
#1760=DIRECTION ( 'NONE',  ( -0.000000000000000000, 0.000000000000000000, 1.000000000000000000 ) ) ;
#1761=EDGE_LOOP ( 'NONE', ( #3456, #1518, #756, #1564 ) ) ;
#1763=VECTOR ( 'NONE', #3197, 1000.000000000000000 ) ;
#1764=ORIENTED_EDGE ( 'NONE', *, *, #4341, .F. ) ;
#1765=CARTESIAN_POINT ( 'NONE',  ( 0.000000000000000000, 0.000000000000000000, 40.00000000000000000 ) ) ;
#1766=ADVANCED_FACE ( 'NONE', ( #1359 ), #5344, .T. ) ;
#1767=FACE_OUTER_BOUND ( 'NONE', #362, .T. ) ;
#1769=CARTESIAN_POINT ( 'NONE',  ( -55.48030965893044453, 45.89047003626346566, 35.00000000000000000 ) ) ;
#1771=AXIS2_PLACEMENT_3D ( 'NONE', #3206, #12, #916 ) ;
#1774=CARTESIAN_POINT ( 'NONE',  ( -11.82353433160510470, 71.60642589802979785, 35.00000000000000000 ) ) ;
#1775=DIRECTION ( 'NONE',  ( -0.4999999999999920619, -0.8660254037844431485, 0.000000000000000000 ) ) ;
#1777=EDGE_CURVE ( 'NONE', #1918, #4090, #4897, .T. ) ;
#1779=B_SPLINE_CURVE_WITH_KNOTS ( 'NONE', 3,
 ( #1705, #2685, #1774, #3606 ),
 .UNSPECIFIED., .F., .F.,
 ( 4, 4 ),
 ( 1.430489624538199204E-17, 0.001907370850886582142 ),
 .UNSPECIFIED. ) ;
#1783=DIRECTION ( 'NONE',  ( 0.7787725926866162496, -0.6273063437270228748, 0.000000000000000000 ) ) ;
#1784=ADVANCED_FACE ( 'NONE', ( #159 ), #1582, .F. ) ;
#1785=DIRECTION ( 'NONE',  ( 1.000000000000000000, 0.000000000000000000, 0.000000000000000000 ) ) ;
#1786=LINE ( 'NONE', #3681, #4033 ) ;
#1787=DIRECTION ( 'NONE',  ( 1.000000000000000000, 0.000000000000000000, 0.000000000000000000 ) ) ;
#1788=EDGE_CURVE ( 'NONE', #3906, #3800, #3130, .T. ) ;
#1790=ORIENTED_EDGE ( 'NONE', *, *, #5419, .F. ) ;
#1791=CARTESIAN_POINT ( 'NONE',  ( -7.182140071210238271E-14, 8.916303653273167033E-14, 35.00000000000000000 ) ) ;
#1792=ORIENTED_EDGE ( 'NONE', *, *, #1318, .T. ) ;
#1794=CARTESIAN_POINT ( 'NONE',  ( 58.45671475544962448, 33.75000000000001421, -35.00000000000000000 ) ) ;
#1795=FACE_OUTER_BOUND ( 'NONE', #1587, .T. ) ;
#1798=VERTEX_POINT ( 'NONE', #1109 ) ;
#1804=CARTESIAN_POINT ( 'NONE',  ( -8.056095891487838412E-14, 1.254589464284425060E-14, -35.00000000000000000 ) ) ;
#1805=ORIENTED_EDGE ( 'NONE', *, *, #2673, .T. ) ;
#1807=CARTESIAN_POINT ( 'NONE',  ( -11.60016251788559849, -72.19966265504864111, 35.04915833130703362 ) ) ;
#1808=EDGE_LOOP ( 'NONE', ( #630, #3406 ) ) ;
#1810=EDGE_CURVE ( 'NONE', #103, #5851, #472, .T. ) ;
#1813=ADVANCED_FACE ( 'NONE', ( #3539 ), #579, .F. ) ;
#1814=ORIENTED_EDGE ( 'NONE', *, *, #1442, .F. ) ;
#1816=VERTEX_POINT ( 'NONE', #2585 ) ;
#1817=DIRECTION ( 'NONE',  ( 1.000000000000000000, 0.000000000000000000, 0.000000000000000000 ) ) ;
#1822=FACE_OUTER_BOUND ( 'NONE', #2280, .T. ) ;
#1823=VECTOR ( 'NONE', #491, 999.9999999999998863 ) ;
#1824=ORIENTED_EDGE ( 'NONE', *, *, #5617, .T. ) ;
#1826=DIRECTION ( 'NONE',  ( 0.000000000000000000, 0.000000000000000000, 1.000000000000000000 ) ) ;
#1827=PLANE ( 'NONE',  #3255 ) ;
#1828=SHAPE_REPRESENTATION_RELATIONSHIP ( 'NONE' , 'NONE' ,  #4975, #2480 ) ;
#1829=VECTOR ( 'NONE', #3742, 1000.000000000000227 ) ;
#1830=CARTESIAN_POINT ( 'NONE',  ( 9.074396217167732814, -58.26942451214393515, -35.00000000000000000 ) ) ;
#1833=AXIS2_PLACEMENT_3D ( 'NONE', #3217, #4708, #2753 ) ;
#1835=VECTOR ( 'NONE', #55, 1000.000000000000000 ) ;
#1837=EDGE_LOOP ( 'NONE', ( #3272, #4682, #483, #1175 ) ) ;
#1838=CARTESIAN_POINT ( 'NONE',  ( 55.48030965893076427, -45.89047003626308197, 35.00000000000000000 ) ) ;
#1839=EDGE_CURVE ( 'NONE', #2060, #5346, #1515, .T. ) ;
#1841=FACE_OUTER_BOUND ( 'NONE', #736, .T. ) ;
#1843=AXIS2_PLACEMENT_3D ( 'NONE', #881, #5575, #3292 ) ;
#1846=EDGE_CURVE ( 'NONE', #3338, #3265, #682, .T. ) ;
#1849=ORIENTED_EDGE ( 'NONE', *, *, #3679, .T. ) ;
#1850=CARTESIAN_POINT ( 'NONE',  ( 57.58482424179643999, 72.37680137756268550, -40.00000000000000000 ) ) ;
#1851=ORIENTED_EDGE ( 'NONE', *, *, #1592, .T. ) ;
#1852=DIRECTION ( 'NONE',  ( 1.000000000000000000, 0.000000000000000000, 0.000000000000000000 ) ) ;
#1853=CARTESIAN_POINT ( 'NONE',  ( -100.0000000000000000, 1.224646799147353217E-14, -39.00000000000002842 ) ) ;
#1854=VECTOR ( 'NONE', #1246, 1000.000000000000000 ) ;
#1855=CARTESIAN_POINT ( 'NONE',  ( 0.000000000000000000, 89.46264649666795776, -79.99999999999998579 ) ) ;
#1856=ORIENTED_EDGE ( 'NONE', *, *, #3921, .T. ) ;
#1857=EDGE_CURVE ( 'NONE', #705, #3262, #5418, .T. ) ;
#1858=FACE_BOUND ( 'NONE', #3383, .T. ) ;
#1859=AXIS2_PLACEMENT_3D ( 'NONE', #5359, #2392, #4282 ) ;
#1860=CARTESIAN_POINT ( 'NONE',  ( -7.182140071210238271E-14, 8.916303653273167033E-14, -35.00000000000000000 ) ) ;
#1864=DIRECTION ( 'NONE',  ( -1.000000000000000000, 0.000000000000000000, 0.000000000000000000 ) ) ;
#1865=DIRECTION ( 'NONE',  ( 1.000000000000000000, 0.000000000000000000, 0.000000000000000000 ) ) ;
#1867=AXIS2_PLACEMENT_3D ( 'NONE', #4906, #1646, #4881 ) ;
#1869=EDGE_CURVE ( 'NONE', #5370, #4211, #1158, .T. ) ;
#1872=ORIENTED_EDGE ( 'NONE', *, *, #4917, .F. ) ;
#1874=ORIENTED_EDGE ( 'NONE', *, *, #4920, .F. ) ;
#1875=CARTESIAN_POINT ( 'NONE',  ( 8.056095891487838412E-14, -1.254589464284425060E-14, -35.00000000000000000 ) ) ;
#1876=ORIENTED_EDGE ( 'NONE', *, *, #1260, .T. ) ;
#1877=DIRECTION ( 'NONE',  ( -1.000000000000000000, 0.000000000000000000, 0.000000000000000000 ) ) ;
#1883=VERTEX_POINT ( 'NONE', #3044 ) ;
#1884=CARTESIAN_POINT ( 'NONE',  ( 0.000000000000000000, 0.000000000000000000, -35.00000000000000000 ) ) ;
#1885=EDGE_CURVE ( 'NONE', #2186, #103, #3012, .T. ) ;
#1887=EDGE_LOOP ( 'NONE', ( #4843, #6138, #1497, #282 ) ) ;
#1888=LINE ( 'NONE', #2829, #5268 ) ;
#1890=ORIENTED_EDGE ( 'NONE', *, *, #2056, .T. ) ;
#1892=CARTESIAN_POINT ( 'NONE',  ( 52.58482424179643289, 72.37680137756268550, -79.99999999999998579 ) ) ;
#1893=EDGE_CURVE ( 'NONE', #1548, #906, #3533, .T. ) ;
#1895=PRODUCT_DEFINITION_SHAPE ( 'NONE', 'NONE',  #313 ) ;
#1896=CARTESIAN_POINT ( 'NONE',  ( -5.114554293134481958E-14, -6.349488965209747807E-14, 35.00000000000000000 ) ) ;
#1898=DIRECTION ( 'NONE',  ( -0.000000000000000000, -0.000000000000000000, -1.000000000000000000 ) ) ;
#1899=CARTESIAN_POINT ( 'NONE',  ( -52.58482424179695158, -72.37680137756228760, -79.99999999999998579 ) ) ;
#1905=ORIENTED_EDGE ( 'NONE', *, *, #749, .T. ) ;
#1906=LINE ( 'NONE', #4785, #1835 ) ;
#1909=CARTESIAN_POINT ( 'NONE',  ( -11.07913919611939058, -71.14248150488579370, 45.00000000000000711 ) ) ;
#1910=CARTESIAN_POINT ( 'NONE',  ( -68.32682326288350794, 26.05379589900699955, 35.04915833130718994 ) ) ;
#1911=EDGE_LOOP ( 'NONE', ( #2794, #5809, #5934, #5629, #3854, #578, #3393, #4503, #2809 ) ) ;
#1912=CYLINDRICAL_SURFACE ( 'NONE', #604, 100.0000000000000000 ) ;
#1913=EDGE_CURVE ( 'NONE', #3466, #1013, #1447, .T. ) ;
#1914=DIRECTION ( 'NONE',  ( 0.7787725926866162496, -0.6273063437270228748, 0.000000000000000000 ) ) ;
#1915=VERTEX_POINT ( 'NONE', #4349 ) ;
#1918=VERTEX_POINT ( 'NONE', #1983 ) ;
#1921=CARTESIAN_POINT ( 'NONE',  ( 0.000000000000000000, 89.46264649666795776, -40.00000000000000000 ) ) ;
#1923=CARTESIAN_POINT ( 'NONE',  ( -52.58482424179536707, 72.37680137756343868, -79.99999999999998579 ) ) ;
#1925=CARTESIAN_POINT ( 'NONE',  ( 0.000000000000000000, 0.000000000000000000, 40.00000000000000000 ) ) ;
#1927=VECTOR ( 'NONE', #424, 1000.000000000000000 ) ;
#1928=EDGE_CURVE ( 'NONE', #2502, #5015, #5324, .T. ) ;
#1929=TOROIDAL_SURFACE ( 'NONE', #4825, 72.00000000000004263, 10.00000000000000000 ) ;
#1930=EDGE_CURVE ( 'NONE', #5851, #103, #2238, .T. ) ;
#1931=VERTEX_POINT ( 'NONE', #347 ) ;
#1933=LINE ( 'NONE', #88, #6040 ) ;
#1935=AXIS2_PLACEMENT_3D ( 'NONE', #5163, #6067, #1787 ) ;
#1937=VECTOR ( 'NONE', #1031, 1000.000000000000000 ) ;
#1938=EDGE_LOOP ( 'NONE', ( #1666, #3495, #1750, #5986, #998, #4596 ) ) ;
#1939=CARTESIAN_POINT ( 'NONE',  ( -74.61196207728360719, -28.86269417393314285, 38.99999999999995737 ) ) ;
#1940=ADVANCED_FACE ( 'NONE', ( #288 ), #4178, .F. ) ;
#1941=VECTOR ( 'NONE', #461, 999.9999999999998863 ) ;
#1943=AXIS2_PLACEMENT_3D ( 'NONE', #34, #5728, #1010 ) ;
#1951=LINE ( 'NONE', #3809, #4218 ) ;
#1953=CARTESIAN_POINT ( 'NONE',  ( -5.114554293134481958E-14, -6.349488965209747807E-14, 35.00000000000000000 ) ) ;
#1954=EDGE_LOOP ( 'NONE', ( #5506, #3572, #2381, #2093 ) ) ;
#1955=DIRECTION ( 'NONE',  ( 1.000000000000000000, 0.000000000000000000, 0.000000000000000000 ) ) ;
#1957=ORIENTED_EDGE ( 'NONE', *, *, #2017, .T. ) ;
#1958=LINE ( 'NONE', #1804, #976 ) ;
#1960=DIRECTION ( 'NONE',  ( 1.000000000000000000, 0.000000000000000000, 0.000000000000000000 ) ) ;
#1961=CARTESIAN_POINT ( 'NONE',  ( -46.52501622030217021, -37.47620048660763103, 35.00000000000000000 ) ) ;
#1965=CIRCLE ( 'NONE', #1661, 9.999999999999996447 ) ;
#1966=AXIS2_PLACEMENT_3D ( 'NONE', #3599, #5577, #3202 ) ;
#1970=CARTESIAN_POINT ( 'NONE',  ( -58.45671475544968843, 33.74999999999987210, -35.00000000000000000 ) ) ;
#1972=EDGE_CURVE ( 'NONE', #4835, #5782, #3620, .T. ) ;
#1974=VERTEX_POINT ( 'NONE', #3256 ) ;
#1975=DIRECTION ( 'NONE',  ( -0.000000000000000000, 0.000000000000000000, 1.000000000000000000 ) ) ;
#1977=ORIENTED_EDGE ( 'NONE', *, *, #1039, .T. ) ;
#1982=ORIENTED_EDGE ( 'NONE', *, *, #6125, .F. ) ;
#1983=CARTESIAN_POINT ( 'NONE',  ( 80.08403291566574467, -27.64547812922912939, -40.00000000000000000 ) ) ;
#1986=DIRECTION ( 'NONE',  ( -0.5000000000000038858, 0.8660254037844362651, 0.000000000000000000 ) ) ;
#1987=VERTEX_POINT ( 'NONE', #3193 ) ;
#1990=EDGE_LOOP ( 'NONE', ( #3199, #3898, #5564, #4576 ) ) ;
#1991=FACE_OUTER_BOUND ( 'NONE', #3011, .T. ) ;
#1992=ORIENTED_EDGE ( 'NONE', *, *, #2439, .T. ) ;
#1996=FACE_OUTER_BOUND ( 'NONE', #4497, .T. ) ;
#1998=VERTEX_POINT ( 'NONE', #2669 ) ;
#1999=ORIENTED_EDGE ( 'NONE', *, *, #2983, .T. ) ;
#2006=EDGE_LOOP ( 'NONE', ( #6106, #1874, #3024, #1381 ) ) ;
#2008=EDGE_CURVE ( 'NONE', #5015, #1165, #3828, .T. ) ;
#2011=ORIENTED_EDGE ( 'NONE', *, *, #4643, .F. ) ;
#2012=DIRECTION ( 'NONE',  ( -1.000000000000000000, 0.000000000000000000, 0.000000000000000000 ) ) ;
#2013=FACE_OUTER_BOUND ( 'NONE', #5397, .T. ) ;
#2014=DIRECTION ( 'NONE',  ( 0.000000000000000000, 0.000000000000000000, 1.000000000000000000 ) ) ;
#2015=EDGE_CURVE ( 'NONE', #656, #404, #5570, .T. ) ;
#2016=CARTESIAN_POINT ( 'NONE',  ( 0.000000000000000000, 0.000000000000000000, 38.99999999999995737 ) ) ;
#2017=EDGE_CURVE ( 'NONE', #747, #2051, #3132, .T. ) ;
#2020=VERTEX_POINT ( 'NONE', #4061 ) ;
#2024=DIRECTION ( 'NONE',  ( 0.5000000000000099920, -0.8660254037844329345, 0.000000000000000000 ) ) ;
#2029=FACE_OUTER_BOUND ( 'NONE', #5417, .T. ) ;
#2030=AXIS2_PLACEMENT_3D ( 'NONE', #4674, #4644, #2804 ) ;
#2031=ORIENTED_EDGE ( 'NONE', *, *, #1323, .T. ) ;
#2036=AXIS2_PLACEMENT_3D ( 'NONE', #5518, #4512, #4580 ) ;
#2038=AXIS2_PLACEMENT_3D ( 'NONE', #3997, #2609, #4086 ) ;
#2041=LINE ( 'NONE', #3941, #607 ) ;
#2043=ORIENTED_EDGE ( 'NONE', *, *, #5626, .F. ) ;
#2044=CARTESIAN_POINT ( 'NONE',  ( -8.056095891487838412E-14, 1.254589464284425060E-14, 35.00000000000000000 ) ) ;
#2046=AXIS2_PLACEMENT_3D ( 'NONE', #4865, #2722, #1756 ) ;
#2048=DIRECTION ( 'NONE',  ( 0.000000000000000000, 0.000000000000000000, 1.000000000000000000 ) ) ;
#2051=VERTEX_POINT ( 'NONE', #410 ) ;
#2054=DIRECTION ( 'NONE',  ( 1.000000000000000000, 0.000000000000000000, 0.000000000000000000 ) ) ;
#2055=DIRECTION ( 'NONE',  ( -0.000000000000000000, -0.000000000000000000, 1.000000000000000000 ) ) ;
#2056=EDGE_CURVE ( 'NONE', #993, #4299, #876, .T. ) ;
#2058=CIRCLE ( 'NONE', #4746, 10.00000000000000355 ) ;
#2059=DIRECTION ( 'NONE',  ( 1.000000000000000000, 0.000000000000000000, 0.000000000000000000 ) ) ;
#2060=VERTEX_POINT ( 'NONE', #3655 ) ;
#2063=DIRECTION ( 'NONE',  ( -1.000000000000000000, 0.000000000000000000, 0.000000000000000000 ) ) ;
#2064=EDGE_CURVE ( 'NONE', #5893, #3309, #1786, .T. ) ;
#2065=VERTEX_POINT ( 'NONE', #2287 ) ;
#2066=FACE_OUTER_BOUND ( 'NONE', #3648, .T. ) ;
#2068=AXIS2_PLACEMENT_3D ( 'NONE', #4722, #478, #2359 ) ;
#2069=ORIENTED_EDGE ( 'NONE', *, *, #4520, .F. ) ;
#2071=VECTOR ( 'NONE', #5274, 1000.000000000000000 ) ;
#2073=VECTOR ( 'NONE', #2378, 1000.000000000000000 ) ;
#2074=FACE_OUTER_BOUND ( 'NONE', #3507, .T. ) ;
#2076=DIRECTION ( 'NONE',  ( 0.000000000000000000, 0.000000000000000000, 1.000000000000000000 ) ) ;
#2078=ORIENTED_EDGE ( 'NONE', *, *, #3761, .T. ) ;
#2080=ORIENTED_EDGE ( 'NONE', *, *, #3266, .F. ) ;
#2081=DIRECTION ( 'NONE',  ( 1.000000000000000000, 0.000000000000000000, 0.000000000000000000 ) ) ;
#2084=DIRECTION ( 'NONE',  ( -1.000000000000000000, 0.000000000000000000, 0.000000000000000000 ) ) ;
#2085=LINE ( 'NONE', #1562, #2481 ) ;
#2088=ORIENTED_EDGE ( 'NONE', *, *, #5192, .F. ) ;
#2089=DIRECTION ( 'NONE',  ( -0.000000000000000000, -0.000000000000000000, 1.000000000000000000 ) ) ;
#2093=ORIENTED_EDGE ( 'NONE', *, *, #1694, .T. ) ;
#2097=ORIENTED_EDGE ( 'NONE', *, *, #5913, .F. ) ;
#2099=CARTESIAN_POINT ( 'NONE',  ( 0.000000000000000000, 0.000000000000000000, 45.00000000000000711 ) ) ;
#2100=CARTESIAN_POINT ( 'NONE',  ( -5.000000000000629718, -89.46264649666795776, -79.99999999999998579 ) ) ;
#2101=VERTEX_POINT ( 'NONE', #2850 ) ;
#2102=CARTESIAN_POINT ( 'NONE',  ( -4.130675435985315210E-14, -1.067806758184287486E-13, -35.00000000000000000 ) ) ;
#2105=LINE ( 'NONE', #1218, #4132 ) ;
#2106=ORIENTED_EDGE ( 'NONE', *, *, #1558, .T. ) ;
#2107=DIRECTION ( 'NONE',  ( 1.000000000000000000, 0.000000000000000000, 0.000000000000000000 ) ) ;
#2109=FACE_OUTER_BOUND ( 'NONE', #3598, .T. ) ;
#2111=DIRECTION ( 'NONE',  ( -0.000000000000000000, -0.000000000000000000, -1.000000000000000000 ) ) ;
#2112=LINE ( 'NONE', #1616, #5162 ) ;
#2113=ORIENTED_EDGE ( 'NONE', *, *, #5682, .T. ) ;
#2114=ORIENTED_EDGE ( 'NONE', *, *, #3542, .F. ) ;
#2117=CARTESIAN_POINT ( 'NONE',  ( 56.07162667343580864, 45.16605674834639217, 45.00000000000000711 ) ) ;
#2120=ORIENTED_EDGE ( 'NONE', *, *, #4908, .T. ) ;
#2121=CARTESIAN_POINT ( 'NONE',  ( 0.000000000000000000, 89.46264649666795776, -79.99999999999998579 ) ) ;
#2123=VERTEX_POINT ( 'NONE', #2388 ) ;
#2124=FACE_OUTER_BOUND ( 'NONE', #5190, .T. ) ;
#2128=VECTOR ( 'NONE', #4485, 1000.000000000000000 ) ;
#2130=FACE_OUTER_BOUND ( 'NONE', #824, .T. ) ;
#2132=VERTEX_POINT ( 'NONE', #3740 ) ;
#2134=APPLICATION_CONTEXT ( 'automotive_design' ) ;
#2135=AXIS2_PLACEMENT_3D ( 'NONE', #346, #5127, #435 ) ;
#2138=AXIS2_PLACEMENT_3D ( 'NONE', #2117, #5501, #775 ) ;
#2140=ORIENTED_EDGE ( 'NONE', *, *, #3040, .F. ) ;
#2141=FACE_OUTER_BOUND ( 'NONE', #1146, .T. ) ;
#2142=ORIENTED_EDGE ( 'NONE', *, *, #334, .T. ) ;
#2143=CARTESIAN_POINT ( 'NONE',  ( 11.33314185117008677, -72.77350886804093477, 35.13717928826310555 ) ) ;
#2144=VECTOR ( 'NONE', #2555, 999.9999999999998863 ) ;
#2145=CYLINDRICAL_SURFACE ( 'NONE', #2661, 5.000000000000004441 ) ;
#2148=FACE_OUTER_BOUND ( 'NONE', #2801, .T. ) ;
#2149=CARTESIAN_POINT ( 'NONE',  ( -80.00000000000000000, 0.000000000000000000, -39.00000000000001421 ) ) ;
#2151=VERTEX_POINT ( 'NONE', #623 ) ;
#2154=CARTESIAN_POINT ( 'NONE',  ( 58.45671475544962448, 33.75000000000001421, 35.00000000000000000 ) ) ;
#2157=DIRECTION ( 'NONE',  ( -0.000000000000000000, 0.000000000000000000, 1.000000000000000000 ) ) ;
#2159=EDGE_LOOP ( 'NONE', ( #5816, #5970, #2478, #4338, #4873 ) ) ;
#2161=EDGE_CURVE ( 'NONE', #2841, #730, #3939, .T. ) ;
#2162=DIRECTION ( 'NONE',  ( -0.000000000000000000, 0.000000000000000000, 1.000000000000000000 ) ) ;
#2164=CARTESIAN_POINT ( 'NONE',  ( -68.32682326288144736, -26.05379589900766035, 35.04915833130703362 ) ) ;
#2167=AXIS2_PLACEMENT_3D ( 'NONE', #5305, #4836, #1369 ) ;
#2168=EDGE_CURVE ( 'NONE', #2218, #132, #1958, .T. ) ;
#2169=CARTESIAN_POINT ( 'NONE',  ( -1.131281550719566266E-13, -1.761763928569765259E-14, 35.00000000000000000 ) ) ;
#2170=EDGE_LOOP ( 'NONE', ( #3479, #2191 ) ) ;
#2171=EDGE_LOOP ( 'NONE', ( #3457, #2981, #449, #1065, #4049, #2080, #3605, #3551 ) ) ;
#2172=VECTOR ( 'NONE', #3462, 1000.000000000000000 ) ;
#2174=VECTOR ( 'NONE', #709, 1000.000000000000114 ) ;
#2177=ADVANCED_FACE ( 'NONE', ( #1991 ), #1648, .F. ) ;
#2178=ORIENTED_EDGE ( 'NONE', *, *, #6011, .T. ) ;
#2179=CARTESIAN_POINT ( 'NONE',  ( -55.71784976887214924, 21.55374571496067304, -35.00000000000000000 ) ) ;
#2180=ORIENTED_EDGE ( 'NONE', *, *, #3841, .T. ) ;
#2181=CARTESIAN_POINT ( 'NONE',  ( 0.000000000000000000, 0.000000000000000000, 35.00000000000000000 ) ) ;
#2182=DIRECTION ( 'NONE',  ( -0.000000000000000000, -0.000000000000000000, -1.000000000000000000 ) ) ;
#2184=FACE_OUTER_BOUND ( 'NONE', #5323, .T. ) ;
#2185=CARTESIAN_POINT ( 'NONE',  ( 0.000000000000000000, 0.000000000000000000, 38.99999999999995737 ) ) ;
#2186=VERTEX_POINT ( 'NONE', #4834 ) ;
#2188=CARTESIAN_POINT ( 'NONE',  ( -9.074396217167167933, -58.26942451214404173, -35.00000000000000000 ) ) ;
#2190=CARTESIAN_POINT ( 'NONE',  ( 0.000000000000000000, 0.000000000000000000, -35.00000000000000000 ) ) ;
#2191=ORIENTED_EDGE ( 'NONE', *, *, #2710, .F. ) ;
#2194=ORIENTED_EDGE ( 'NONE', *, *, #5522, .F. ) ;
#2195=FACE_OUTER_BOUND ( 'NONE', #5178, .T. ) ;
#2200=EDGE_CURVE ( 'NONE', #836, #2604, #4440, .T. ) ;
#2202=VERTEX_POINT ( 'NONE', #4874 ) ;
#2203=CARTESIAN_POINT ( 'NONE',  ( -80.99999999999998579, 0.000000000000000000, -40.00000000000000000 ) ) ;
#2204=VERTEX_POINT ( 'NONE', #3700 ) ;
#2205=DIRECTION ( 'NONE',  ( 1.000000000000000000, 0.000000000000000000, 0.000000000000000000 ) ) ;
#2207=DIRECTION ( 'NONE',  ( -0.8660254037844339337, -0.5000000000000079936, 0.000000000000000000 ) ) ;
#2208=EDGE_CURVE ( 'NONE', #2569, #1495, #3344, .T. ) ;
#2211=ORIENTED_EDGE ( 'NONE', *, *, #1200, .T. ) ;
#2213=DIRECTION ( 'NONE',  ( 0.000000000000000000, 0.000000000000000000, 1.000000000000000000 ) ) ;
#2214=LINE ( 'NONE', #4168, #2958 ) ;
#2218=VERTEX_POINT ( 'NONE', #5016 ) ;
#2221=CARTESIAN_POINT ( 'NONE',  ( -8.056095891487838412E-14, 1.254589464284425060E-14, 35.00000000000000000 ) ) ;
#2222=CARTESIAN_POINT ( 'NONE',  ( 11.07913919612032316, -71.14248150488565159, 45.00000000000000711 ) ) ;
#2223=VERTEX_POINT ( 'NONE', #679 ) ;
#2227=CARTESIAN_POINT ( 'NONE',  ( 80.00000000000000000, 9.797174393178826052E-15, -39.00000000000001421 ) ) ;
#2230=EDGE_CURVE ( 'NONE', #3051, #3466, #4948, .T. ) ;
#2232=EDGE_CURVE ( 'NONE', #5114, #4690, #261, .T. ) ;
#2234=DIRECTION ( 'NONE',  ( -0.000000000000000000, 0.000000000000000000, 1.000000000000000000 ) ) ;
#2236=AXIS2_PLACEMENT_3D ( 'NONE', #3837, #4853, #4340 ) ;
#2237=DIRECTION ( 'NONE',  ( 1.000000000000000000, 0.000000000000000000, 0.000000000000000000 ) ) ;
#2238=CIRCLE ( 'NONE', #2046, 5.000000000000004441 ) ;
#2239=VERTEX_POINT ( 'NONE', #3978 ) ;
#2240=PLANE ( 'NONE',  #5258 ) ;
#2242=CARTESIAN_POINT ( 'NONE',  ( -80.08403291566614257, -27.64547812922793923, -79.99999999999998579 ) ) ;
#2243=DIRECTION ( 'NONE',  ( -0.6273063437270329779, 0.7787725926866080339, 0.000000000000000000 ) ) ;
#2244=ORIENTED_EDGE ( 'NONE', *, *, #5192, .T. ) ;
#2249=ORIENTED_EDGE ( 'NONE', *, *, #4446, .T. ) ;
#2252=DIRECTION ( 'NONE',  ( 1.000000000000000000, 0.000000000000000000, 0.000000000000000000 ) ) ;
#2253=DIRECTION ( 'NONE',  ( -0.000000000000000000, -0.000000000000000000, 1.000000000000000000 ) ) ;
#2256=CIRCLE ( 'NONE', #5551, 72.00000000000004263 ) ;
#2257=CARTESIAN_POINT ( 'NONE',  ( -1.630640067418198669E-13, 67.50000000000002842, 35.00000000000000000 ) ) ;
#2261=VERTEX_POINT ( 'NONE', #2562 ) ;
#2265=CARTESIAN_POINT ( 'NONE',  ( -47.58482424179695158, -72.37680137756228760, 40.00000000000000000 ) ) ;
#2266=CARTESIAN_POINT ( 'NONE',  ( 54.99999999999999289, 6.349087922075113966E-13, 35.00000000000000000 ) ) ;
#2268=PLANE ( 'NONE',  #2638 ) ;
#2270=VECTOR ( 'NONE', #4345, 1000.000000000000000 ) ;
#2271=CARTESIAN_POINT ( 'NONE',  ( 68.69027832784067300, -26.57196568621440491, 35.00000000000000000 ) ) ;
#2272=VERTEX_POINT ( 'NONE', #2646 ) ;
#2273=DIRECTION ( 'NONE',  ( 0.1538769332794418798, -0.9880900209011901358, 0.000000000000000000 ) ) ;
#2274=CARTESIAN_POINT ( 'NONE',  ( 46.52501622030217021, 37.47620048660763103, 35.00000000000000000 ) ) ;
#2280=EDGE_LOOP ( 'NONE', ( #5885, #799, #1647, #2561 ) ) ;
#2282=CARTESIAN_POINT ( 'NONE',  ( 0.000000000000000000, 0.000000000000000000, 35.00000000000000000 ) ) ;
#2283=ORIENTED_EDGE ( 'NONE', *, *, #1006, .F. ) ;
#2284=EDGE_CURVE ( 'NONE', #15, #4405, #3057, .T. ) ;
#2285=CARTESIAN_POINT ( 'NONE',  ( -85.08403291566612836, -27.64547812922793923, -79.99999999999998579 ) ) ;
#2286=ADVANCED_FACE ( 'NONE', ( #2141 ), #3109, .F. ) ;
#2287=CARTESIAN_POINT ( 'NONE',  ( -12.49999999999999822, -67.50000000000000000, -35.00000000000000000 ) ) ;
#2288=CARTESIAN_POINT ( 'NONE',  ( -7.182140071210238271E-14, 8.916303653273167033E-14, -35.00000000000000000 ) ) ;
#2292=ORIENTED_EDGE ( 'NONE', *, *, #1928, .F. ) ;
#2293=CARTESIAN_POINT ( 'NONE',  ( -6.247143215332724651E-13, -89.46264649666795776, 40.00000000000000000 ) ) ;
#2296=DIRECTION ( 'NONE',  ( 0.000000000000000000, 0.000000000000000000, 1.000000000000000000 ) ) ;
#2302=CARTESIAN_POINT ( 'NONE',  ( 1.131281550719567528E-13, 1.761763928569687004E-14, 35.00000000000000000 ) ) ;
#2303=CARTESIAN_POINT ( 'NONE',  ( 58.45671475544992290, -33.74999999999945999, -35.00000000000000000 ) ) ;
#2308=ORIENTED_EDGE ( 'NONE', *, *, #3198, .T. ) ;
#2310=CARTESIAN_POINT ( 'NONE',  ( 56.10121673609980064, -46.04269404270027621, 35.00000000000000000 ) ) ;
#2318=EDGE_CURVE ( 'NONE', #5138, #5202, #2105, .T. ) ;
#2319=DIRECTION ( 'NONE',  ( 0.000000000000000000, 0.000000000000000000, -1.000000000000000000 ) ) ;
#2321=DIRECTION ( 'NONE',  ( -0.1538769332794418798, 0.9880900209011901358, 0.000000000000000000 ) ) ;
#2326=CIRCLE ( 'NONE', #5820, 72.00000000000004263 ) ;
#2329=FACE_BOUND ( 'NONE', #4907, .T. ) ;
#2332=VECTOR ( 'NONE', #941, 1000.000000000000000 ) ;
#2333=ORIENTED_EDGE ( 'NONE', *, *, #635, .T. ) ;
#2335=CARTESIAN_POINT ( 'NONE',  ( 55.00000000000024158, -21.27605460799916770, 35.00000000000000000 ) ) ;
#2337=CARTESIAN_POINT ( 'NONE',  ( -55.00000000000010658, 21.27605460799956205, 35.00000000000000000 ) ) ;
#2338=VECTOR ( 'NONE', #819, 1000.000000000000114 ) ;
#2342=AXIS2_PLACEMENT_3D ( 'NONE', #4635, #3141, #4131 ) ;
#2343=AXIS2_PLACEMENT_3D ( 'NONE', #5785, #4886, #2512 ) ;
#2346=VERTEX_POINT ( 'NONE', #2179 ) ;
#2347=DIRECTION ( 'NONE',  ( 0.000000000000000000, 0.000000000000000000, 1.000000000000000000 ) ) ;
#2348=AXIS2_PLACEMENT_3D ( 'NONE', #2525, #1607, #1132 ) ;
#2349=EDGE_LOOP ( 'NONE', ( #2078, #3913, #3960, #648 ) ) ;
#2350=FACE_OUTER_BOUND ( 'NONE', #1585, .T. ) ;
#2354=DIRECTION ( 'NONE',  ( 0.000000000000000000, 0.000000000000000000, 1.000000000000000000 ) ) ;
#2356=LINE ( 'NONE', #3876, #2270 ) ;
#2357=VECTOR ( 'NONE', #2375, 1000.000000000000000 ) ;
#2358=ORIENTED_EDGE ( 'NONE', *, *, #4339, .F. ) ;
#2359=DIRECTION ( 'NONE',  ( 1.000000000000000000, 0.000000000000000000, 0.000000000000000000 ) ) ;
#2360=ORIENTED_EDGE ( 'NONE', *, *, #1737, .F. ) ;
#2361=DIRECTION ( 'NONE',  ( -0.000000000000000000, -0.000000000000000000, 1.000000000000000000 ) ) ;
#2362=CARTESIAN_POINT ( 'NONE',  ( -12.31015466235495026, -79.04720167209526949, 35.00000000000000000 ) ) ;
#2364=PLANE ( 'NONE',  #3812 ) ;
#2368=VECTOR ( 'NONE', #5106, 1000.000000000000114 ) ;
#2370=VERTEX_POINT ( 'NONE', #2227 ) ;
#2371=CIRCLE ( 'NONE', #4558, 5.000000000000004441 ) ;
#2372=ORIENTED_EDGE ( 'NONE', *, *, #2232, .F. ) ;
#2373=LINE ( 'NONE', #1498, #1102 ) ;
#2375=DIRECTION ( 'NONE',  ( -0.000000000000000000, -0.000000000000000000, -1.000000000000000000 ) ) ;
#2378=DIRECTION ( 'NONE',  ( -0.000000000000000000, -0.000000000000000000, -1.000000000000000000 ) ) ;
#2381=ORIENTED_EDGE ( 'NONE', *, *, #4137, .T. ) ;
#2384=DIRECTION ( 'NONE',  ( 0.000000000000000000, 0.000000000000000000, 1.000000000000000000 ) ) ;
#2388=CARTESIAN_POINT ( 'NONE',  ( 4.999999999999380940, -89.46264649666795776, 40.00000000000000000 ) ) ;
#2392=DIRECTION ( 'NONE',  ( 0.000000000000000000, 0.000000000000000000, 1.000000000000000000 ) ) ;
#2393=VERTEX_POINT ( 'NONE', #4129 ) ;
#2394=CARTESIAN_POINT ( 'NONE',  ( 6.314393452555577824E-13, -67.50000000000002842, 35.00000000000000000 ) ) ;
#2398=FACE_OUTER_BOUND ( 'NONE', #3403, .T. ) ;
#2399=ORIENTED_EDGE ( 'NONE', *, *, #2427, .T. ) ;
#2400=CARTESIAN_POINT ( 'NONE',  ( 58.45671475544992290, -33.74999999999945999, 35.00000000000000000 ) ) ;
#2403=ORIENTED_EDGE ( 'NONE', *, *, #3155, .T. ) ;
#2404=FACE_OUTER_BOUND ( 'NONE', #5902, .T. ) ;
#2406=CARTESIAN_POINT ( 'NONE',  ( -2.941541598353333735E-14, 7.604078429494112756E-14, 35.00000000000000000 ) ) ;
#2408=ADVANCED_FACE ( 'NONE', ( #3687 ), #1357, .F. ) ;
#2409=DIRECTION ( 'NONE',  ( 1.000000000000000000, 0.000000000000000000, 0.000000000000000000 ) ) ;
#2415=EDGE_LOOP ( 'NONE', ( #4852, #3503, #3974, #4421 ) ) ;
#2419=DIRECTION ( 'NONE',  ( -0.1538769332794359679, -0.9880900209011910240, 0.000000000000000000 ) ) ;
#2423=DIRECTION ( 'NONE',  ( -1.000000000000000000, 0.000000000000000000, 0.000000000000000000 ) ) ;
#2424=ORIENTED_EDGE ( 'NONE', *, *, #5419, .T. ) ;
#2427=EDGE_CURVE ( 'NONE', #5773, #3865, #480, .T. ) ;
#2430=AXIS2_PLACEMENT_3D ( 'NONE', #4524, #1655, #4468 ) ;
#2432=FACE_OUTER_BOUND ( 'NONE', #4602, .T. ) ;
#2433=CARTESIAN_POINT ( 'NONE',  ( 2.941541598353386116E-14, -7.604078429494091299E-14, -35.00000000000000000 ) ) ;
#2434=DIRECTION ( 'NONE',  ( -0.000000000000000000, -0.000000000000000000, -1.000000000000000000 ) ) ;
#2437=VECTOR ( 'NONE', #2835, 1000.000000000000000 ) ;
#2438=AXIS2_PLACEMENT_3D ( 'NONE', #1517, #2048, #1133 ) ;
#2439=EDGE_CURVE ( 'NONE', #2239, #2261, #852, .T. ) ;
#2440=EDGE_LOOP ( 'NONE', ( #2524, #1617, #4970, #4165 ) ) ;
#2442=CARTESIAN_POINT ( 'NONE',  ( -12.31015466235523981, 79.04720167209522685, -35.00000000000000000 ) ) ;
#2444=AXIS2_PLACEMENT_3D ( 'NONE', #2724, #4626, #2757 ) ;
#2445=VERTEX_POINT ( 'NONE', #441 ) ;
#2446=DIRECTION ( 'NONE',  ( -1.000000000000000000, 0.000000000000000000, 0.000000000000000000 ) ) ;
#2448=EDGE_CURVE ( 'NONE', #193, #2445, #937, .T. ) ;
#2450=AXIS2_PLACEMENT_3D ( 'NONE', #5862, #3480, #4953 ) ;
#2455=DIRECTION ( 'NONE',  ( 0.9326495259660445569, 0.3607836771741652626, 0.000000000000000000 ) ) ;
#2457=ORIENTED_EDGE ( 'NONE', *, *, #6077, .F. ) ;
#2458=DIRECTION ( 'NONE',  ( 0.000000000000000000, 0.000000000000000000, 1.000000000000000000 ) ) ;
#2459=CLOSED_SHELL ( 'NONE', ( #5594, #4685, #5213, #3638, #5801, #1015, #3802, #3307, #4856, #5905, #1251, #2885, #1766, #5867, #4770, #5495, #5667, #933, #5738, #3721, #1528, #3465, #5717, #4175, #6058, #4509, #4065, #4709, #3986, #209, #1291, #1701, #3085, #2408, #512, #2286, #2818, #926, #5407, #1599, #4028, #4294, #5300, #4106, #3764, #5751, #1482, #1940, #433, #6087, #612, #3123, #4415, #5449, #3961, #1813, #2508, #1235, #1292, #6099, #5414, #357, #4624, #4715, #5838, #5709, #4344, #1434, #1784, #1059, #4060, #1559, #3345, #5912, #977, #5625, #4488, #3987, #2623, #5598, #3163, #5441, #3223, #426, #1709, #3952, #3095, #4332, #4926, #391, #4169, #2177, #5385, #4710, #3683, #3678, #3877 ) ) ;
#2460=DIRECTION ( 'NONE',  ( -0.7071067811865573427, 8.659560562355053653E-17, 0.7071067811865378028 ) ) ;
#2461=CARTESIAN_POINT ( 'NONE',  ( -67.48246767247790956, -25.10212255632935197, 35.00000000000000000 ) ) ;
#2462=ORIENTED_EDGE ( 'NONE', *, *, #5521, .T. ) ;
#2464=CIRCLE ( 'NONE', #5055, 10.00000000000000355 ) ;
#2466=ORIENTED_EDGE ( 'NONE', *, *, #5338, .T. ) ;
#2467=DIRECTION ( 'NONE',  ( -0.000000000000000000, -0.000000000000000000, 1.000000000000000000 ) ) ;
#2468=VERTEX_POINT ( 'NONE', #4158 ) ;
#2469=PLANE ( 'NONE',  #302 ) ;
#2471=DIRECTION ( 'NONE',  ( -0.000000000000000000, 0.000000000000000000, 1.000000000000000000 ) ) ;
#2473=CIRCLE ( 'NONE', #3460, 72.00000000000004263 ) ;
#2474=CYLINDRICAL_SURFACE ( 'NONE', #3658, 5.000000000000004441 ) ;
#2477=AXIS2_PLACEMENT_3D ( 'NONE', #3052, #1557, #5464 ) ;
#2478=ORIENTED_EDGE ( 'NONE', *, *, #2600, .T. ) ;
#2480=ADVANCED_BREP_SHAPE_REPRESENTATION ( '', ( #4196, #73 ), #5734 ) ;
#2481=VECTOR ( 'NONE', #4935, 1000.000000000000114 ) ;
#2486=CARTESIAN_POINT ( 'NONE',  ( -58.45671475544962448, -33.75000000000001421, -35.00000000000000000 ) ) ;
#2487=VECTOR ( 'NONE', #4934, 1000.000000000000000 ) ;
#2489=VERTEX_POINT ( 'NONE', #4212 ) ;
#2491=EDGE_CURVE ( 'NONE', #2502, #4858, #5263, .T. ) ;
#2493=CARTESIAN_POINT ( 'NONE',  ( -56.07162667343580864, -45.16605674834639217, 45.00000000000000711 ) ) ;
#2495=CARTESIAN_POINT ( 'NONE',  ( 90.08403291566594362, 27.64547812922851833, -79.99999999999998579 ) ) ;
#2496=DIRECTION ( 'NONE',  ( -0.000000000000000000, -0.000000000000000000, -1.000000000000000000 ) ) ;
#2498=EDGE_LOOP ( 'NONE', ( #5681, #2946 ) ) ;
#2502=VERTEX_POINT ( 'NONE', #1850 ) ;
#2503=LINE ( 'NONE', #3980, #4352 ) ;
#2504=LINE ( 'NONE', #3574, #3562 ) ;
#2507=DIRECTION ( 'NONE',  ( 0.000000000000000000, 0.000000000000000000, -1.000000000000000000 ) ) ;
#2508=ADVANCED_FACE ( 'NONE', ( #3200 ), #6070, .F. ) ;
#2509=ORIENTED_EDGE ( 'NONE', *, *, #5532, .F. ) ;
#2512=DIRECTION ( 'NONE',  ( 1.000000000000000000, 0.000000000000000000, 0.000000000000000000 ) ) ;
#2513=EDGE_LOOP ( 'NONE', ( #5670, #4265, #4157, #33 ) ) ;
#2516=EDGE_LOOP ( 'NONE', ( #2178, #4875, #2672, #861, #42 ) ) ;
#2518=EDGE_CURVE ( 'NONE', #3250, #670, #6096, .T. ) ;
#2520=EDGE_CURVE ( 'NONE', #5804, #1288, #389, .T. ) ;
#2523=DIRECTION ( 'NONE',  ( -0.000000000000000000, -0.000000000000000000, 1.000000000000000000 ) ) ;
#2524=ORIENTED_EDGE ( 'NONE', *, *, #1260, .F. ) ;
#2525=CARTESIAN_POINT ( 'NONE',  ( -27.50000000000000355, -47.63139720814412215, 35.00000000000000000 ) ) ;
#2526=CARTESIAN_POINT ( 'NONE',  ( -67.92475106770288562, -25.56373185532869741, 35.00000000000000000 ) ) ;
#2535=CARTESIAN_POINT ( 'NONE',  ( 52.58482424179591419, -72.37680137756305498, -79.99999999999998579 ) ) ;
#2536=ORIENTED_EDGE ( 'NONE', *, *, #2903, .F. ) ;
#2537=CARTESIAN_POINT ( 'NONE',  ( 80.08403291566592941, 27.64547812922851833, -79.99999999999998579 ) ) ;
#2538=DIRECTION ( 'NONE',  ( 0.1538769332794418798, -0.9880900209011900248, 0.000000000000000000 ) ) ;
#2541=ORIENTED_EDGE ( 'NONE', *, *, #2788, .F. ) ;
#2544=ORIENTED_EDGE ( 'NONE', *, *, #4564, .T. ) ;
#2545=STYLED_ITEM('',(#6198),#4196);
#2547=AXIS2_PLACEMENT_3D ( 'NONE', #2394, #3294, #4215 ) ;
#2548=B_SPLINE_CURVE_WITH_KNOTS ( 'NONE', 3,
 ( #2461, #2526, #2164, #4447 ),
 .UNSPECIFIED., .F., .F.,
 ( 4, 4 ),
 ( 3.469446951953614189E-18, 0.001907370850883722234 ),
 .UNSPECIFIED. ) ;
#2550=AXIS2_PLACEMENT_3D ( 'NONE', #3738, #3218, #6120 ) ;
#2555=DIRECTION ( 'NONE',  ( 0.1538769332794359124, 0.9880900209011910240, 0.000000000000000000 ) ) ;
#2557=DIRECTION ( 'NONE',  ( -0.000000000000000000, -0.000000000000000000, -1.000000000000000000 ) ) ;
#2561=ORIENTED_EDGE ( 'NONE', *, *, #4643, .T. ) ;
#2562=CARTESIAN_POINT ( 'NONE',  ( 74.61196207728410457, -28.86269417393182479, -35.00000000000000000 ) ) ;
#2563=EDGE_LOOP ( 'NONE', ( #2544, #3778, #5924, #830, #5907, #3430, #3724, #2541, #2509 ) ) ;
#2565=CARTESIAN_POINT ( 'NONE',  ( 85.08403291566592941, 27.64547812922851833, -40.00000000000000000 ) ) ;
#2566=LINE ( 'NONE', #5843, #2128 ) ;
#2568=LINE ( 'NONE', #4967, #1577 ) ;
#2569=VERTEX_POINT ( 'NONE', #3844 ) ;
#2570=VECTOR ( 'NONE', #2595, 1000.000000000000000 ) ;
#2572=CARTESIAN_POINT ( 'NONE',  ( -55.71784976887420271, -21.55374571496209057, -35.00000000000000000 ) ) ;
#2574=EDGE_LOOP ( 'NONE', ( #2120, #1872, #2069, #4139 ) ) ;
#2579=AXIS2_PLACEMENT_3D ( 'NONE', #2181, #1726, #1244 ) ;
#2580=CARTESIAN_POINT ( 'NONE',  ( 0.000000000000000000, 0.000000000000000000, -40.00000000000000000 ) ) ;
#2581=VECTOR ( 'NONE', #981, 1000.000000000000000 ) ;
#2583=DIRECTION ( 'NONE',  ( -0.000000000000000000, -0.000000000000000000, 1.000000000000000000 ) ) ;
#2584=ORIENTED_EDGE ( 'NONE', *, *, #4407, .F. ) ;
#2585=CARTESIAN_POINT ( 'NONE',  ( 57.35713647666955950, -46.20154318182373032, -35.00000000000000000 ) ) ;
#2587=DIRECTION ( 'NONE',  ( 0.9880900209011910240, -0.1538769332794358846, 0.000000000000000000 ) ) ;
#2590=DIRECTION ( 'NONE',  ( -0.000000000000000000, -0.000000000000000000, -1.000000000000000000 ) ) ;
#2595=DIRECTION ( 'NONE',  ( -0.000000000000000000, -0.000000000000000000, 1.000000000000000000 ) ) ;
#2596=CARTESIAN_POINT ( 'NONE',  ( -6.247143215332724651E-13, -89.46264649666795776, -79.99999999999998579 ) ) ;
#2597=CARTESIAN_POINT ( 'NONE',  ( 0.000000000000000000, 0.000000000000000000, 40.00000000000000000 ) ) ;
#2598=ORIENTED_EDGE ( 'NONE', *, *, #4446, .F. ) ;
#2600=EDGE_CURVE ( 'NONE', #5916, #3596, #701, .T. ) ;
#2603=DIRECTION ( 'NONE',  ( 1.000000000000000000, 0.000000000000000000, 0.000000000000000000 ) ) ;
#2604=VERTEX_POINT ( 'NONE', #5230 ) ;
#2605=CARTESIAN_POINT ( 'NONE',  ( -46.52501622030217021, -37.47620048660763103, -35.00000000000000000 ) ) ;
#2607=ORIENTED_EDGE ( 'NONE', *, *, #708, .F. ) ;
#2609=DIRECTION ( 'NONE',  ( -0.000000000000000000, -0.000000000000000000, -1.000000000000000000 ) ) ;
#2611=LINE ( 'NONE', #5979, #3923 ) ;
#2613=ORIENTED_EDGE ( 'NONE', *, *, #409, .F. ) ;
#2616=ORIENTED_EDGE ( 'NONE', *, *, #2600, .F. ) ;
#2617=CARTESIAN_POINT ( 'NONE',  ( 58.45671475544921947, 33.75000000000068212, 35.00000000000000000 ) ) ;
#2619=LINE ( 'NONE', #5805, #1743 ) ;
#2621=CARTESIAN_POINT ( 'NONE',  ( 27.50000000000000355, 47.63139720814412215, 35.00000000000000000 ) ) ;
#2622=CARTESIAN_POINT ( 'NONE',  ( 68.69027832784067300, -26.57196568621440491, -35.00000000000000000 ) ) ;
#2623=ADVANCED_FACE ( 'NONE', ( #1513 ), #3463, .F. ) ;
#2624=EDGE_LOOP ( 'NONE', ( #2823, #2952, #2424, #1234 ) ) ;
#2628=ORIENTED_EDGE ( 'NONE', *, *, #4138, .F. ) ;
#2629=EDGE_CURVE ( 'NONE', #3966, #2204, #5957, .T. ) ;
#2630=CARTESIAN_POINT ( 'NONE',  ( 46.52501622030442974, -37.47620048660870395, -35.00000000000000000 ) ) ;
#2631=EDGE_CURVE ( 'NONE', #2705, #5491, #2857, .T. ) ;
#2634=FACE_BOUND ( 'NONE', #1273, .T. ) ;
#2635=AXIS2_PLACEMENT_3D ( 'NONE', #1508, #1975, #4751 ) ;
#2636=EDGE_CURVE ( 'NONE', #1013, #2727, #4555, .T. ) ;
#2637=VECTOR ( 'NONE', #3973, 1000.000000000000114 ) ;
#2638=AXIS2_PLACEMENT_3D ( 'NONE', #6074, #1702, #2708 ) ;
#2639=DIRECTION ( 'NONE',  ( 0.000000000000000000, 0.000000000000000000, 1.000000000000000000 ) ) ;
#2642=AXIS2_PLACEMENT_3D ( 'NONE', #5549, #6044, #517 ) ;
#2644=CIRCLE ( 'NONE', #65, 5.000000000000004441 ) ;
#2645=EDGE_LOOP ( 'NONE', ( #43, #4535 ) ) ;
#2646=CARTESIAN_POINT ( 'NONE',  ( -45.92560378283290845, 36.99336990414408888, 35.00000000000000000 ) ) ;
#2648=PLANE ( 'NONE',  #1367 ) ;
#2651=DIRECTION ( 'NONE',  ( -1.000000000000000000, 0.000000000000000000, 0.000000000000000000 ) ) ;
#2653=VECTOR ( 'NONE', #2321, 1000.000000000000114 ) ;
#2654=ORIENTED_EDGE ( 'NONE', *, *, #3407, .T. ) ;
#2660=DIRECTION ( 'NONE',  ( -0.000000000000000000, -0.000000000000000000, -1.000000000000000000 ) ) ;
#2661=AXIS2_PLACEMENT_3D ( 'NONE', #210, #2055, #1115 ) ;
#2664=DIRECTION ( 'NONE',  ( 1.000000000000000000, 0.000000000000000000, 0.000000000000000000 ) ) ;
#2665=EDGE_CURVE ( 'NONE', #3865, #5773, #3065, .T. ) ;
#2667=CARTESIAN_POINT ( 'NONE',  ( 6.314393452555577824E-13, -67.50000000000002842, 35.00000000000000000 ) ) ;
#2669=CARTESIAN_POINT ( 'NONE',  ( -90.08403291566554572, 27.64547812922971914, -40.00000000000000000 ) ) ;
#2670=AXIS2_PLACEMENT_3D ( 'NONE', #2963, #4931, #3486 ) ;
#2672=ORIENTED_EDGE ( 'NONE', *, *, #1415, .F. ) ;
#2673=EDGE_CURVE ( 'NONE', #5910, #1915, #2748, .T. ) ;
#2676=ORIENTED_EDGE ( 'NONE', *, *, #4466, .F. ) ;
#2677=DIRECTION ( 'NONE',  ( -1.000000000000000000, 0.000000000000000000, 0.000000000000000000 ) ) ;
#2678=ORIENTED_EDGE ( 'NONE', *, *, #1810, .F. ) ;
#2679=FACE_OUTER_BOUND ( 'NONE', #3947, .T. ) ;
#2680=DIRECTION ( 'NONE',  ( -1.000000000000000000, 0.000000000000000000, 0.000000000000000000 ) ) ;
#2681=DIRECTION ( 'NONE',  ( 1.000000000000000000, 0.000000000000000000, 0.000000000000000000 ) ) ;
#2683=DIRECTION ( 'NONE',  ( 0.3607836771741718684, -0.9326495259660421144, 0.000000000000000000 ) ) ;
#2684=ORIENTED_EDGE ( 'NONE', *, *, #3752, .F. ) ;
#2685=CARTESIAN_POINT ( 'NONE',  ( -11.60016251788669450, 72.19966265505019010, 35.04915833130718994 ) ) ;
#2690=B_SPLINE_CURVE_WITH_KNOTS ( 'NONE', 3,
 ( #4653, #1753, #1807, #2812 ),
 .UNSPECIFIED., .F., .F.,
 ( 4, 4 ),
 ( 0.000000000000000000, 0.001907370850883695563 ),
 .UNSPECIFIED. ) ;
#2692=ORIENTED_EDGE ( 'NONE', *, *, #1450, .F. ) ;
#2694=FACE_OUTER_BOUND ( 'NONE', #3560, .T. ) ;
#2695=DIRECTION ( 'NONE',  ( 0.000000000000000000, -0.000000000000000000, -1.000000000000000000 ) ) ;
#2696=EDGE_CURVE ( 'NONE', #4711, #2774, #2041, .T. ) ;
#2697=EDGE_CURVE ( 'NONE', #4858, #1165, #2985, .T. ) ;
#2700=ORIENTED_EDGE ( 'NONE', *, *, #635, .F. ) ;
#2705=VERTEX_POINT ( 'NONE', #390 ) ;
#2706=CYLINDRICAL_SURFACE ( 'NONE', #5555, 100.0000000000000000 ) ;
#2708=DIRECTION ( 'NONE',  ( 0.5000000000000101030, -0.8660254037844328234, 0.000000000000000000 ) ) ;
#2710=EDGE_CURVE ( 'NONE', #1308, #2828, #798, .T. ) ;
#2711=LINE ( 'NONE', #2271, #1475 ) ;
#2713=DIRECTION ( 'NONE',  ( 1.000000000000000000, 0.000000000000000000, 0.000000000000000000 ) ) ;
#2714=DIRECTION ( 'NONE',  ( -0.000000000000000000, -0.000000000000000000, -1.000000000000000000 ) ) ;
#2718=ORIENTED_EDGE ( 'NONE', *, *, #5876, .T. ) ;
#2720=DIRECTION ( 'NONE',  ( 1.000000000000000000, 0.000000000000000000, 0.000000000000000000 ) ) ;
#2721=LINE ( 'NONE', #408, #5933 ) ;
#2722=DIRECTION ( 'NONE',  ( 0.000000000000000000, 0.000000000000000000, 1.000000000000000000 ) ) ;
#2724=CARTESIAN_POINT ( 'NONE',  ( 0.000000000000000000, 0.000000000000000000, 38.99999999999995737 ) ) ;
#2725=AXIS2_PLACEMENT_3D ( 'NONE', #6015, #3635, #5054 ) ;
#2727=VERTEX_POINT ( 'NONE', #5672 ) ;
#2730=ORIENTED_EDGE ( 'NONE', *, *, #4531, .F. ) ;
#2731=CARTESIAN_POINT ( 'NONE',  ( 11.60016251788720076, -72.19966265505010483, 35.04915833130718994 ) ) ;
#2732=CIRCLE ( 'NONE', #5234, 81.00000000000004263 ) ;
#2733=LINE ( 'NONE', #2266, #3741 ) ;
#2734=EDGE_CURVE ( 'NONE', #4773, #132, #5554, .T. ) ;
#2737=AXIS2_PLACEMENT_3D ( 'NONE', #2844, #3252, #4201 ) ;
#2739=DIRECTION ( 'NONE',  ( 0.9326495259660420034, 0.3607836771741718129, 0.000000000000000000 ) ) ;
#2740=ORIENTED_EDGE ( 'NONE', *, *, #9, .F. ) ;
#2743=EDGE_CURVE ( 'NONE', #2101, #3175, #2711, .T. ) ;
#2748=B_SPLINE_CURVE_WITH_KNOTS ( 'NONE', 3,
 ( #32, #1910, #157, #5860 ),
 .UNSPECIFIED., .F., .F.,
 ( 4, 4 ),
 ( 3.469446951953614189E-18, 0.001907370850886582576 ),
 .UNSPECIFIED. ) ;
#2753=DIRECTION ( 'NONE',  ( 1.000000000000000000, 0.000000000000000000, 0.000000000000000000 ) ) ;
#2756=VECTOR ( 'NONE', #2182, 1000.000000000000000 ) ;
#2757=DIRECTION ( 'NONE',  ( 1.000000000000000000, 0.000000000000000000, 0.000000000000000000 ) ) ;
#2758=CIRCLE ( 'NONE', #501, 5.000000000000004441 ) ;
#2760=AXIS2_PLACEMENT_3D ( 'NONE', #1921, #1464, #552 ) ;
#2762=ORIENTED_EDGE ( 'NONE', *, *, #723, .T. ) ;
#2764=VECTOR ( 'NONE', #1486, 1000.000000000000000 ) ;
#2765=EDGE_LOOP ( 'NONE', ( #549, #4663, #2999, #713 ) ) ;
#2766=CARTESIAN_POINT ( 'NONE',  ( -12.50000000000155431, 67.50000000000002842, 35.00000000000000000 ) ) ;
#2768=ORIENTED_EDGE ( 'NONE', *, *, #5007, .T. ) ;
#2770=VECTOR ( 'NONE', #4010, 1000.000000000000000 ) ;
#2771=CARTESIAN_POINT ( 'NONE',  ( -12.50000000000155431, 67.50000000000002842, -35.00000000000000000 ) ) ;
#2774=VERTEX_POINT ( 'NONE', #1397 ) ;
#2780=EDGE_CURVE ( 'NONE', #3800, #1013, #1965, .T. ) ;
#2781=EDGE_CURVE ( 'NONE', #3309, #2774, #4048, .T. ) ;
#2782=CARTESIAN_POINT ( 'NONE',  ( 0.000000000000000000, 0.000000000000000000, 45.00000000000000711 ) ) ;
#2785=FACE_OUTER_BOUND ( 'NONE', #4067, .T. ) ;
#2786=ORIENTED_EDGE ( 'NONE', *, *, #5150, .T. ) ;
#2788=EDGE_CURVE ( 'NONE', #4001, #2218, #1573, .T. ) ;
#2790=DIRECTION ( 'NONE',  ( -1.000000000000000000, 0.000000000000000000, 0.000000000000000000 ) ) ;
#2794=ORIENTED_EDGE ( 'NONE', *, *, #4408, .T. ) ;
#2795=DIRECTION ( 'NONE',  ( 0.000000000000000000, 0.000000000000000000, 1.000000000000000000 ) ) ;
#2796=DIRECTION ( 'NONE',  ( -1.000000000000000000, 0.000000000000000000, 0.000000000000000000 ) ) ;
#2798=ORIENTED_EDGE ( 'NONE', *, *, #99, .F. ) ;
#2799=CARTESIAN_POINT ( 'NONE',  ( 0.000000000000000000, 89.46264649666795776, 40.00000000000000000 ) ) ;
#2801=EDGE_LOOP ( 'NONE', ( #4632, #3688, #4240, #5147, #1226, #842, #1764, #5222, #2740 ) ) ;
#2804=DIRECTION ( 'NONE',  ( 1.000000000000000000, 0.000000000000000000, 0.000000000000000000 ) ) ;
#2806=DIRECTION ( 'NONE',  ( -0.000000000000000000, -0.000000000000000000, -1.000000000000000000 ) ) ;
#2807=EDGE_CURVE ( 'NONE', #5943, #3250, #4223, .T. ) ;
#2809=ORIENTED_EDGE ( 'NONE', *, *, #5211, .F. ) ;
#2812=CARTESIAN_POINT ( 'NONE',  ( -11.33314185116896589, -72.77350886803867525, 35.13717928826270054 ) ) ;
#2813=EDGE_CURVE ( 'NONE', #3566, #4690, #3239, .T. ) ;
#2817=CARTESIAN_POINT ( 'NONE',  ( 0.000000000000000000, 0.000000000000000000, -35.00000000000000000 ) ) ;
#2818=ADVANCED_FACE ( 'NONE', ( #1822 ), #1307, .F. ) ;
#2821=ORIENTED_EDGE ( 'NONE', *, *, #2788, .T. ) ;
#2822=DIRECTION ( 'NONE',  ( 0.7787725926866119197, -0.6273063437270283149, 0.000000000000000000 ) ) ;
#2823=ORIENTED_EDGE ( 'NONE', *, *, #5766, .T. ) ;
#2824=PLANE ( 'NONE',  #3234 ) ;
#2825=PLANE ( 'NONE',  #5154 ) ;
#2826=CIRCLE ( 'NONE', #6018, 4.999999999999990230 ) ;
#2828=VERTEX_POINT ( 'NONE', #4640 ) ;
#2829=CARTESIAN_POINT ( 'NONE',  ( -8.056095891487838412E-14, 1.254589464284425060E-14, -35.00000000000000000 ) ) ;
#2833=ORIENTED_EDGE ( 'NONE', *, *, #3236, .F. ) ;
#2834=CARTESIAN_POINT ( 'NONE',  ( 0.000000000000000000, 0.000000000000000000, -35.00000000000000000 ) ) ;
#2835=DIRECTION ( 'NONE',  ( -0.000000000000000000, -0.000000000000000000, 1.000000000000000000 ) ) ;
#2838=LINE ( 'NONE', #1406, #2073 ) ;
#2841=VERTEX_POINT ( 'NONE', #2771 ) ;
#2844=CARTESIAN_POINT ( 'NONE',  ( -85.08403291566612836, -27.64547812922793923, -79.99999999999998579 ) ) ;
#2846=VERTEX_POINT ( 'NONE', #335 ) ;
#2847=CARTESIAN_POINT ( 'NONE',  ( 74.61196207728339402, 28.86269417393366865, 35.00000000000000000 ) ) ;
#2850=CARTESIAN_POINT ( 'NONE',  ( 68.69027832784067300, -26.57196568621440491, 35.13717928826310555 ) ) ;
#2851=EDGE_CURVE ( 'NONE', #2186, #2998, #2758, .T. ) ;
#2852=EDGE_CURVE ( 'NONE', #2204, #3836, #1334, .T. ) ;
#2857=LINE ( 'NONE', #3448, #1100 ) ;
#2862=DIRECTION ( 'NONE',  ( 1.000000000000000000, 0.000000000000000000, 0.000000000000000000 ) ) ;
#2865=VECTOR ( 'NONE', #1280, 1000.000000000000000 ) ;
#2869=CARTESIAN_POINT ( 'NONE',  ( 9.192833548570215285, 59.02994620157096506, 35.00000000000000000 ) ) ;
#2870=DIRECTION ( 'NONE',  ( -0.000000000000000000, -0.000000000000000000, 1.000000000000000000 ) ) ;
#2874=CARTESIAN_POINT ( 'NONE',  ( -9.074396217167327805, 58.26942451214400620, 35.00000000000000000 ) ) ;
#2875=DIRECTION ( 'NONE',  ( 0.7787725926866080339, 0.6273063437270329779, 0.000000000000000000 ) ) ;
#2876=AXIS2_PLACEMENT_3D ( 'NONE', #5013, #5282, #1501 ) ;
#2877=EDGE_LOOP ( 'NONE', ( #5038, #1363, #4418, #5329, #5489, #5064 ) ) ;
#2881=EDGE_LOOP ( 'NONE', ( #1792, #4913, #4429, #4442 ) ) ;
#2882=CARTESIAN_POINT ( 'NONE',  ( 4.130675435985391572E-14, 1.067806758184284836E-13, -35.00000000000000000 ) ) ;
#2885=ADVANCED_FACE ( 'NONE', ( #4689 ), #1365, .T. ) ;
#2888=ORIENTED_EDGE ( 'NONE', *, *, #5471, .T. ) ;
#2889=CARTESIAN_POINT ( 'NONE',  ( 100.0000000000000000, 1.224646799147353217E-14, -39.00000000000002842 ) ) ;
#2891=VERTEX_POINT ( 'NONE', #4209 ) ;
#2898=ORIENTED_EDGE ( 'NONE', *, *, #3427, .T. ) ;
#2899=CARTESIAN_POINT ( 'NONE',  ( 0.000000000000000000, 0.000000000000000000, 35.00000000000000000 ) ) ;
#2900=CARTESIAN_POINT ( 'NONE',  ( -52.58482424179536707, 72.37680137756343868, -79.99999999999998579 ) ) ;
#2902=CARTESIAN_POINT ( 'NONE',  ( 90.08403291566575888, -27.64547812922912939, 40.00000000000000000 ) ) ;
#2903=EDGE_CURVE ( 'NONE', #670, #5794, #201, .T. ) ;
#2905=ORIENTED_EDGE ( 'NONE', *, *, #1669, .F. ) ;
#2909=ORIENTED_EDGE ( 'NONE', *, *, #5338, .F. ) ;
#2915=ORIENTED_EDGE ( 'NONE', *, *, #5502, .T. ) ;
#2916=CARTESIAN_POINT ( 'NONE',  ( -54.99999999999990052, -21.27605460800010206, 35.00000000000000000 ) ) ;
#2917=CARTESIAN_POINT ( 'NONE',  ( -57.35713647666923976, 46.20154318182412112, 35.00000000000000000 ) ) ;
#2919=FACE_BOUND ( 'NONE', #3187, .T. ) ;
#2923=AXIS2_PLACEMENT_3D ( 'NONE', #222, #2157, #4051 ) ;
#2925=CARTESIAN_POINT ( 'NONE',  ( 55.48030965893076427, -45.89047003626308197, 35.00000000000000000 ) ) ;
#2926=EDGE_CURVE ( 'NONE', #1883, #4004, #1299, .T. ) ;
#2927=CYLINDRICAL_SURFACE ( 'NONE', #5031, 4.999999999999997335 ) ;
#2928=CARTESIAN_POINT ( 'NONE',  ( -100.0000000000000000, 0.000000000000000000, 40.00000000000000000 ) ) ;
#2932=AXIS2_PLACEMENT_3D ( 'NONE', #3114, #5552, #855 ) ;
#2934=ORIENTED_EDGE ( 'NONE', *, *, #1625, .F. ) ;
#2938=CARTESIAN_POINT ( 'NONE',  ( -27.50000000000010303, 47.63139720814406530, 35.00000000000000000 ) ) ;
#2939=AXIS2_PLACEMENT_3D ( 'NONE', #786, #5040, #4499 ) ;
#2942=LINE ( 'NONE', #603, #4528 ) ;
#2943=CIRCLE ( 'NONE', #1344, 80.99999999999998579 ) ;
#2946=ORIENTED_EDGE ( 'NONE', *, *, #1266, .T. ) ;
#2952=ORIENTED_EDGE ( 'NONE', *, *, #5708, .F. ) ;
#2953=DIRECTION ( 'NONE',  ( -0.000000000000000000, -0.000000000000000000, 1.000000000000000000 ) ) ;
#2954=CARTESIAN_POINT ( 'NONE',  ( 0.000000000000000000, 0.000000000000000000, 35.00000000000000000 ) ) ;
#2956=DIRECTION ( 'NONE',  ( -1.000000000000000000, 0.000000000000000000, 0.000000000000000000 ) ) ;
#2957=ORIENTED_EDGE ( 'NONE', *, *, #4383, .T. ) ;
#2958=VECTOR ( 'NONE', #4675, 1000.000000000000000 ) ;
#2960=ORIENTED_EDGE ( 'NONE', *, *, #4239, .F. ) ;
#2961=DIRECTION ( 'NONE',  ( -0.000000000000000000, -0.000000000000000000, -1.000000000000000000 ) ) ;
#2962=ORIENTED_EDGE ( 'NONE', *, *, #2743, .F. ) ;
#2963=CARTESIAN_POINT ( 'NONE',  ( 0.000000000000000000, 0.000000000000000000, -35.00000000000000000 ) ) ;
#2964=CARTESIAN_POINT ( 'NONE',  ( -6.247143215332724651E-13, -89.46264649666795776, -40.00000000000000000 ) ) ;
#2965=AXIS2_PLACEMENT_3D ( 'NONE', #5085, #6100, #5988 ) ;
#2967=DIRECTION ( 'NONE',  ( 1.000000000000000000, 0.000000000000000000, 0.000000000000000000 ) ) ;
#2971=AXIS2_PLACEMENT_3D ( 'NONE', #1892, #79, #3759 ) ;
#2974=CIRCLE ( 'NONE', #5865, 12.50000000000000178 ) ;
#2976=CARTESIAN_POINT ( 'NONE',  ( 11.33314185116896589, 72.77350886803867525, 35.13717928826270054 ) ) ;
#2978=EDGE_CURVE ( 'NONE', #4044, #1046, #5470, .T. ) ;
#2979=AXIS2_PLACEMENT_3D ( 'NONE', #454, #530, #5745 ) ;
#2981=ORIENTED_EDGE ( 'NONE', *, *, #3761, .F. ) ;
#2983=EDGE_CURVE ( 'NONE', #4283, #656, #5663, .T. ) ;
#2985=LINE ( 'NONE', #4895, #4351 ) ;
#2987=CARTESIAN_POINT ( 'NONE',  ( -80.08403291566554572, 27.64547812922971914, -79.99999999999998579 ) ) ;
#2988=CYLINDRICAL_SURFACE ( 'NONE', #3930, 12.50000000000139089 ) ;
#2989=FACE_OUTER_BOUND ( 'NONE', #4502, .T. ) ;
#2991=EDGE_LOOP ( 'NONE', ( #1101, #6069 ) ) ;
#2993=DIRECTION ( 'NONE',  ( 0.9326495259660518844, -0.3607836771741464998, 0.000000000000000000 ) ) ;
#2994=CARTESIAN_POINT ( 'NONE',  ( -58.45671475544946816, -33.75000000000027711, 35.00000000000000000 ) ) ;
#2996=DIRECTION ( 'NONE',  ( -1.000000000000000000, 0.000000000000000000, 0.000000000000000000 ) ) ;
#2997=FACE_OUTER_BOUND ( 'NONE', #4188, .T. ) ;
#2998=VERTEX_POINT ( 'NONE', #5293 ) ;
#2999=ORIENTED_EDGE ( 'NONE', *, *, #1869, .T. ) ;
#3000=LINE ( 'NONE', #5847, #4514 ) ;
#3002=DIRECTION ( 'NONE',  ( 1.000000000000000000, 0.000000000000000000, 0.000000000000000000 ) ) ;
#3003=EDGE_CURVE ( 'NONE', #4984, #2020, #1007, .T. ) ;
#3005=CARTESIAN_POINT ( 'NONE',  ( 9.074396217167732814, -58.26942451214393515, 35.00000000000000000 ) ) ;
#3007=ORIENTED_EDGE ( 'NONE', *, *, #2813, .T. ) ;
#3009=EDGE_CURVE ( 'NONE', #5996, #3996, #2356, .T. ) ;
#3011=EDGE_LOOP ( 'NONE', ( #2194, #3284, #5472, #5789, #256 ) ) ;
#3012=LINE ( 'NONE', #2495, #3240 ) ;
#3014=CARTESIAN_POINT ( 'NONE',  ( -9.192833548570002122, 59.02994620156853500, 35.00000000000000000 ) ) ;
#3018=ORIENTED_EDGE ( 'NONE', *, *, #5759, .F. ) ;
#3020=CARTESIAN_POINT ( 'NONE',  ( 57.35713647666955950, -46.20154318182373032, 35.00000000000000000 ) ) ;
#3022=LINE ( 'NONE', #1645, #1336 ) ;
#3023=CARTESIAN_POINT ( 'NONE',  ( 55.71784976887403928, 21.55374571496248137, 35.00000000000000000 ) ) ;
#3024=ORIENTED_EDGE ( 'NONE', *, *, #5184, .T. ) ;
#3025=LINE ( 'NONE', #2537, #4205 ) ;
#3026=CARTESIAN_POINT ( 'NONE',  ( 90.08403291566594362, 27.64547812922851833, 40.00000000000000000 ) ) ;
#3027=CARTESIAN_POINT ( 'NONE',  ( 0.000000000000000000, 0.000000000000000000, -35.00000000000000000 ) ) ;
#3030=EDGE_CURVE ( 'NONE', #5498, #3338, #3409, .T. ) ;
#3031=CARTESIAN_POINT ( 'NONE',  ( -11.33314185116896589, -72.77350886803867525, 35.13717928826270054 ) ) ;
#3033=AXIS2_PLACEMENT_3D ( 'NONE', #2257, #4154, #878 ) ;
#3034=ORIENTED_EDGE ( 'NONE', *, *, #4992, .T. ) ;
#3035=DIRECTION ( 'NONE',  ( -0.3607836771741531612, -0.9326495259660493309, 0.000000000000000000 ) ) ;
#3037=VECTOR ( 'NONE', #3770, 999.9999999999998863 ) ;
#3038=AXIS2_PLACEMENT_3D ( 'NONE', #3801, #5316, #1062 ) ;
#3040=EDGE_CURVE ( 'NONE', #1013, #4784, #4252, .T. ) ;
#3043=ORIENTED_EDGE ( 'NONE', *, *, #4844, .T. ) ;
#3044=CARTESIAN_POINT ( 'NONE',  ( 62.30180741492923602, -50.18450749816189216, 38.99999999999995737 ) ) ;
#3045=AXIS2_PLACEMENT_3D ( 'NONE', #5168, #5665, #6042 ) ;
#3047=EDGE_CURVE ( 'NONE', #4773, #5881, #1104, .T. ) ;
#3049=ORIENTED_EDGE ( 'NONE', *, *, #1558, .F. ) ;
#3051=VERTEX_POINT ( 'NONE', #3776 ) ;
#3052=CARTESIAN_POINT ( 'NONE',  ( 0.000000000000000000, -67.50000000000000000, -35.00000000000000000 ) ) ;
#3055=DIRECTION ( 'NONE',  ( -0.000000000000000000, -0.000000000000000000, -1.000000000000000000 ) ) ;
#3057=B_SPLINE_CURVE_WITH_KNOTS ( 'NONE', 3,
 ( #3484, #797, #3571, #1610 ),
 .UNSPECIFIED., .F., .F.,
 ( 4, 4 ),
 ( 0.000000000000000000, 0.001907370850883704887 ),
 .UNSPECIFIED. ) ;
#3058=DIRECTION ( 'NONE',  ( 0.000000000000000000, 0.000000000000000000, 1.000000000000000000 ) ) ;
#3060=VECTOR ( 'NONE', #4728, 1000.000000000000000 ) ;
#3061=ORIENTED_EDGE ( 'NONE', *, *, #5708, .T. ) ;
#3064=( NAMED_UNIT ( * ) SI_UNIT ( $, .STERADIAN. ) SOLID_ANGLE_UNIT ( ) );
#3065=CIRCLE ( 'NONE', #2068, 5.000000000000004441 ) ;
#3067=CYLINDRICAL_SURFACE ( 'NONE', #53, 5.000000000000003553 ) ;
#3068=CIRCLE ( 'NONE', #197, 12.50000000000000000 ) ;
#3070=AXIS2_PLACEMENT_3D ( 'NONE', #3815, #5733, #1955 ) ;
#3072=CYLINDRICAL_SURFACE ( 'NONE', #2038, 12.49999999999999822 ) ;
#3073=CIRCLE ( 'NONE', #3857, 12.50000000000138733 ) ;
#3078=ORIENTED_EDGE ( 'NONE', *, *, #6077, .T. ) ;
#3082=DIRECTION ( 'NONE',  ( -0.000000000000000000, -0.000000000000000000, -1.000000000000000000 ) ) ;
#3084=CARTESIAN_POINT ( 'NONE',  ( -57.58482424179535997, 72.37680137756343868, 40.00000000000000000 ) ) ;
#3085=ADVANCED_FACE ( 'NONE', ( #5250 ), #4271, .F. ) ;
#3086=CARTESIAN_POINT ( 'NONE',  ( -68.69027832784050247, 26.57196568621489163, -35.00000000000000000 ) ) ;
#3087=SHAPE_DEFINITION_REPRESENTATION ( #1895, #4975 ) ;
#3089=CARTESIAN_POINT ( 'NONE',  ( 0.000000000000000000, 0.000000000000000000, 40.00000000000000000 ) ) ;
#3090=DIRECTION ( 'NONE',  ( -1.000000000000000000, 0.000000000000000000, 0.000000000000000000 ) ) ;
#3091=ORIENTED_EDGE ( 'NONE', *, *, #3874, .F. ) ;
#3094=PLANE ( 'NONE',  #577 ) ;
#3095=ADVANCED_FACE ( 'NONE', ( #5680 ), #4232, .F. ) ;
#3097=FACE_OUTER_BOUND ( 'NONE', #415, .T. ) ;
#3100=VERTEX_POINT ( 'NONE', #558 ) ;
#3101=DIRECTION ( 'NONE',  ( 1.000000000000000000, 0.000000000000000000, 0.000000000000000000 ) ) ;
#3103=DIRECTION ( 'NONE',  ( -0.000000000000000000, -0.000000000000000000, -1.000000000000000000 ) ) ;
#3104=ORIENTED_EDGE ( 'NONE', *, *, #3615, .F. ) ;
#3108=ORIENTED_EDGE ( 'NONE', *, *, #1155, .T. ) ;
#3109=CYLINDRICAL_SURFACE ( 'NONE', #283, 12.49999999999999645 ) ;
#3110=EDGE_LOOP ( 'NONE', ( #912, #2962, #1400, #4291, #2403 ) ) ;
#3112=LINE ( 'NONE', #1676, #4860 ) ;
#3114=CARTESIAN_POINT ( 'NONE',  ( -6.247143215332724651E-13, -89.46264649666795776, -79.99999999999998579 ) ) ;
#3117=ORIENTED_EDGE ( 'NONE', *, *, #3994, .T. ) ;
#3118=CARTESIAN_POINT ( 'NONE',  ( -62.30180741492890206, 50.18450749816231848, 38.99999999999995737 ) ) ;
#3120=CARTESIAN_POINT ( 'NONE',  ( -11.07913919611982223, 71.14248150488573685, 45.00000000000000711 ) ) ;
#3123=ADVANCED_FACE ( 'NONE', ( #1435 ), #5214, .F. ) ;
#3126=CARTESIAN_POINT ( 'NONE',  ( 55.00000000000024158, -21.27605460799916770, 35.00000000000000000 ) ) ;
#3127=FACE_BOUND ( 'NONE', #1808, .T. ) ;
#3128=CIRCLE ( 'NONE', #1330, 5.000000000000004441 ) ;
#3129=( LENGTH_UNIT ( ) NAMED_UNIT ( * ) SI_UNIT ( .MILLI., .METRE. ) );
#3130=B_SPLINE_CURVE_WITH_KNOTS ( 'NONE', 3,
 ( #4443, #617, #200, #5890 ),
 .UNSPECIFIED., .F., .F.,
 ( 4, 4 ),
 ( 0.000000000000000000, 0.001907370850883699249 ),
 .UNSPECIFIED. ) ;
#3131=VECTOR ( 'NONE', #4267, 1000.000000000000227 ) ;
#3132=LINE ( 'NONE', #5593, #4026 ) ;
#3134=ORIENTED_EDGE ( 'NONE', *, *, #4145, .T. ) ;
#3137=VECTOR ( 'NONE', #3152, 1000.000000000000000 ) ;
#3141=DIRECTION ( 'NONE',  ( 0.000000000000000000, 0.000000000000000000, 1.000000000000000000 ) ) ;
#3145=LINE ( 'NONE', #3205, #960 ) ;
#3148=ORIENTED_EDGE ( 'NONE', *, *, #848, .T. ) ;
#3149=DIRECTION ( 'NONE',  ( -0.9880900209011901358, -0.1538769332794418798, 0.000000000000000000 ) ) ;
#3150=CARTESIAN_POINT ( 'NONE',  ( -67.48246767247790956, -25.10212255632935197, 35.00000000000000000 ) ) ;
#3152=DIRECTION ( 'NONE',  ( -0.8660254037844385966, 0.5000000000000001110, 0.000000000000000000 ) ) ;
#3153=VECTOR ( 'NONE', #1093, 1000.000000000000000 ) ;
#3155=EDGE_CURVE ( 'NONE', #1077, #3262, #2112, .T. ) ;
#3161=LINE ( 'NONE', #3530, #2338 ) ;
#3162=VECTOR ( 'NONE', #4932, 1000.000000000000000 ) ;
#3163=ADVANCED_FACE ( 'NONE', ( #3514 ), #4255, .T. ) ;
#3164=PLANE ( 'NONE',  #170 ) ;
#3165=AXIS2_PLACEMENT_3D ( 'NONE', #4671, #2683, #2739 ) ;
#3166=AXIS2_PLACEMENT_3D ( 'NONE', #4103, #6020, #3670 ) ;
#3167=CARTESIAN_POINT ( 'NONE',  ( 4.130675435985391572E-14, 1.067806758184284836E-13, 35.00000000000000000 ) ) ;
#3170=EDGE_CURVE ( 'NONE', #1681, #5243, #1201, .T. ) ;
#3171=CIRCLE ( 'NONE', #2979, 10.00000000000000178 ) ;
#3175=VERTEX_POINT ( 'NONE', #2622 ) ;
#3176=DIRECTION ( 'NONE',  ( -0.000000000000000000, -0.000000000000000000, -1.000000000000000000 ) ) ;
#3177=CARTESIAN_POINT ( 'NONE',  ( 0.000000000000000000, -67.50000000000000000, 35.00000000000000000 ) ) ;
#3180=CARTESIAN_POINT ( 'NONE',  ( -11.33314185116896589, -72.77350886803867525, 35.00000000000000000 ) ) ;
#3181=ORIENTED_EDGE ( 'NONE', *, *, #1893, .F. ) ;
#3182=DIRECTION ( 'NONE',  ( 0.000000000000000000, 0.000000000000000000, 1.000000000000000000 ) ) ;
#3183=CARTESIAN_POINT ( 'NONE',  ( -12.49999999999999822, -67.50000000000000000, 35.00000000000000000 ) ) ;
#3187=EDGE_LOOP ( 'NONE', ( #2678, #1082 ) ) ;
#3190=DIRECTION ( 'NONE',  ( 0.000000000000000000, 0.000000000000000000, 1.000000000000000000 ) ) ;
#3192=DIRECTION ( 'NONE',  ( -0.1538769332794358846, -0.9880900209011910240, 0.000000000000000000 ) ) ;
#3193=CARTESIAN_POINT ( 'NONE',  ( -55.71784976887214924, 21.55374571496067304, 35.00000000000000000 ) ) ;
#3194=EDGE_CURVE ( 'NONE', #2828, #1308, #4054, .T. ) ;
#3195=CARTESIAN_POINT ( 'NONE',  ( 52.58482424179643289, 72.37680137756268550, -79.99999999999998579 ) ) ;
#3196=UNCERTAINTY_MEASURE_WITH_UNIT (LENGTH_MEASURE( 1.000000000000000082E-05 ), #3129, 'distance_accuracy_value', 'NONE');
#3197=DIRECTION ( 'NONE',  ( -0.000000000000000000, -0.000000000000000000, -1.000000000000000000 ) ) ;
#3198=EDGE_CURVE ( 'NONE', #5202, #37, #2085, .T. ) ;
#3199=ORIENTED_EDGE ( 'NONE', *, *, #5532, .T. ) ;
#3200=FACE_OUTER_BOUND ( 'NONE', #1124, .T. ) ;
#3202=DIRECTION ( 'NONE',  ( -1.000000000000000000, 0.000000000000000000, 0.000000000000000000 ) ) ;
#3205=CARTESIAN_POINT ( 'NONE',  ( -1.131281550719566266E-13, -1.761763928569765259E-14, 35.00000000000000000 ) ) ;
#3206=CARTESIAN_POINT ( 'NONE',  ( 5.114554293134526134E-14, 6.349488965209711204E-14, 35.00000000000000000 ) ) ;
#3207=DIRECTION ( 'NONE',  ( -1.000000000000000000, 0.000000000000000000, 0.000000000000000000 ) ) ;
#3210=CARTESIAN_POINT ( 'NONE',  ( -46.52501622030417394, 37.47620048660903080, 35.00000000000000000 ) ) ;
#3211=FACE_OUTER_BOUND ( 'NONE', #2349, .T. ) ;
#3217=CARTESIAN_POINT ( 'NONE',  ( 0.000000000000000000, 0.000000000000000000, 40.00000000000000000 ) ) ;
#3218=DIRECTION ( 'NONE',  ( 0.000000000000000000, 0.000000000000000000, 1.000000000000000000 ) ) ;
#3219=DIRECTION ( 'NONE',  ( -0.7071067811865524577, 0.000000000000000000, -0.7071067811865426878 ) ) ;
#3221=LINE ( 'NONE', #1384, #6121 ) ;
#3223=ADVANCED_FACE ( 'NONE', ( #4997 ), #1170, .F. ) ;
#3230=ORIENTED_EDGE ( 'NONE', *, *, #21, .T. ) ;
#3231=FACE_OUTER_BOUND ( 'NONE', #5403, .T. ) ;
#3232=CIRCLE ( 'NONE', #4831, 12.50000000000138556 ) ;
#3233=CARTESIAN_POINT ( 'NONE',  ( -80.99999999999998579, 0.000000000000000000, -40.00000000000000000 ) ) ;
#3234=AXIS2_PLACEMENT_3D ( 'NONE', #1884, #4185, #1852 ) ;
#3235=FACE_OUTER_BOUND ( 'NONE', #2574, .T. ) ;
#3236=EDGE_CURVE ( 'NONE', #4835, #2202, #508, .T. ) ;
#3238=CONICAL_SURFACE ( 'NONE', #4433, 80.00000000000000000, 0.7853981633974482790 ) ;
#3239=LINE ( 'NONE', #1860, #5863 ) ;
#3240=VECTOR ( 'NONE', #4002, 1000.000000000000000 ) ;
#3242=DIRECTION ( 'NONE',  ( -0.9880900209011901358, -0.1538769332794418798, 0.000000000000000000 ) ) ;
#3243=CARTESIAN_POINT ( 'NONE',  ( -1.630640067418198669E-13, 67.50000000000002842, -35.00000000000000000 ) ) ;
#3244=DIRECTION ( 'NONE',  ( 0.9326495259660445569, 0.3607836771741652626, 0.000000000000000000 ) ) ;
#3247=EDGE_CURVE ( 'NONE', #5574, #1077, #4463, .T. ) ;
#3250=VERTEX_POINT ( 'NONE', #2149 ) ;
#3252=DIRECTION ( 'NONE',  ( -0.000000000000000000, -0.000000000000000000, 1.000000000000000000 ) ) ;
#3254=DIRECTION ( 'NONE',  ( -0.000000000000000000, -0.000000000000000000, 1.000000000000000000 ) ) ;
#3255=AXIS2_PLACEMENT_3D ( 'NONE', #5610, #2243, #4645 ) ;
#3256=CARTESIAN_POINT ( 'NONE',  ( 9.192833548570416013, -59.02994620156847105, -35.00000000000000000 ) ) ;
#3262=VERTEX_POINT ( 'NONE', #144 ) ;
#3264=CIRCLE ( 'NONE', #4871, 5.000000000000004441 ) ;
#3265=VERTEX_POINT ( 'NONE', #3580 ) ;
#3266=EDGE_CURVE ( 'NONE', #2891, #3996, #2568, .T. ) ;
#3267=DIRECTION ( 'NONE',  ( -1.154631945610162960E-14, 1.000000000000000000, 0.000000000000000000 ) ) ;
#3268=ORIENTED_EDGE ( 'NONE', *, *, #1839, .T. ) ;
#3270=AXIS2_PLACEMENT_3D ( 'NONE', #3825, #4230, #557 ) ;
#3272=ORIENTED_EDGE ( 'NONE', *, *, #1777, .F. ) ;
#3273=ORIENTED_EDGE ( 'NONE', *, *, #1228, .T. ) ;
#3275=EDGE_CURVE ( 'NONE', #3523, #4211, #3264, .T. ) ;
#3276=LINE ( 'NONE', #5180, #4717 ) ;
#3277=CARTESIAN_POINT ( 'NONE',  ( -2.941541598353333735E-14, 7.604078429494112756E-14, -35.00000000000000000 ) ) ;
#3278=DIRECTION ( 'NONE',  ( -0.000000000000000000, -0.000000000000000000, -1.000000000000000000 ) ) ;
#3280=DIRECTION ( 'NONE',  ( 0.1538769332794359124, 0.9880900209011910240, 0.000000000000000000 ) ) ;
#3281=ORIENTED_EDGE ( 'NONE', *, *, #1450, .T. ) ;
#3282=EDGE_CURVE ( 'NONE', #1523, #2841, #3922, .T. ) ;
#3284=ORIENTED_EDGE ( 'NONE', *, *, #3535, .T. ) ;
#3286=VERTEX_POINT ( 'NONE', #5375 ) ;
#3287=DIRECTION ( 'NONE',  ( 0.000000000000000000, 0.000000000000000000, 1.000000000000000000 ) ) ;
#3290=DIRECTION ( 'NONE',  ( -0.9880900209011910240, 0.1538769332794358846, 0.000000000000000000 ) ) ;
#3292=DIRECTION ( 'NONE',  ( -0.9326495259660518844, 0.3607836771741465554, 0.000000000000000000 ) ) ;
#3294=DIRECTION ( 'NONE',  ( 0.000000000000000000, 0.000000000000000000, 1.000000000000000000 ) ) ;
#3297=VERTEX_POINT ( 'NONE', #3023 ) ;
#3299=DIRECTION ( 'NONE',  ( 0.6273063437270283149, 0.7787725926866120307, -0.000000000000000000 ) ) ;
#3303=DIRECTION ( 'NONE',  ( -0.000000000000000000, -0.000000000000000000, 1.000000000000000000 ) ) ;
#3304=CARTESIAN_POINT ( 'NONE',  ( 0.000000000000000000, 0.000000000000000000, 0.000000000000000000 ) ) ;
#3307=ADVANCED_FACE ( 'NONE', ( #2997 ), #655, .F. ) ;
#3309=VERTEX_POINT ( 'NONE', #3636 ) ;
#3312=CARTESIAN_POINT ( 'NONE',  ( 0.000000000000000000, 0.000000000000000000, 38.99999999999995737 ) ) ;
#3313=ORIENTED_EDGE ( 'NONE', *, *, #4445, .F. ) ;
#3317=LINE ( 'NONE', #379, #1829 ) ;
#3321=DIRECTION ( 'NONE',  ( 1.000000000000000000, 0.000000000000000000, 0.000000000000000000 ) ) ;
#3323=DIRECTION ( 'NONE',  ( 0.000000000000000000, -0.000000000000000000, -1.000000000000000000 ) ) ;
#3327=VECTOR ( 'NONE', #5945, 1000.000000000000000 ) ;
#3328=ORIENTED_EDGE ( 'NONE', *, *, #2200, .T. ) ;
#3329=EDGE_LOOP ( 'NONE', ( #3490, #3346, #2730, #5702, #183, #1685, #616, #3985, #3034, #2957, #2140, #1073, #4093, #1640, #3420, #4031 ) ) ;
#3330=CARTESIAN_POINT ( 'NONE',  ( 9.192833548570215285, 59.02994620157096506, 35.00000000000000000 ) ) ;
#3332=CIRCLE ( 'NONE', #4117, 5.000000000000004441 ) ;
#3333=CARTESIAN_POINT ( 'NONE',  ( 2.941541598353386116E-14, -7.604078429494091299E-14, -35.00000000000000000 ) ) ;
#3334=CIRCLE ( 'NONE', #2343, 80.00000000000000000 ) ;
#3335=FACE_OUTER_BOUND ( 'NONE', #3329, .T. ) ;
#3336=VECTOR ( 'NONE', #4656, 999.9999999999998863 ) ;
#3338=VERTEX_POINT ( 'NONE', #5880 ) ;
#3339=ORIENTED_EDGE ( 'NONE', *, *, #2008, .F. ) ;
#3342=DIRECTION ( 'NONE',  ( 1.000000000000000000, 0.000000000000000000, 0.000000000000000000 ) ) ;
#3343=EDGE_CURVE ( 'NONE', #3966, #5881, #4762, .T. ) ;
#3344=CIRCLE ( 'NONE', #1751, 12.49999999999999822 ) ;
#3345=ADVANCED_FACE ( 'NONE', ( #4608 ), #3666, .F. ) ;
#3346=ORIENTED_EDGE ( 'NONE', *, *, #4341, .T. ) ;
#3347=CARTESIAN_POINT ( 'NONE',  ( -52.58482424179695158, -72.37680137756228760, -40.00000000000000000 ) ) ;
#3352=AXIS2_PLACEMENT_3D ( 'NONE', #1794, #5603, #4667 ) ;
#3354=ORIENTED_EDGE ( 'NONE', *, *, #3529, .F. ) ;
#3355=EDGE_CURVE ( 'NONE', #3286, #1252, #2974, .T. ) ;
#3356=DIRECTION ( 'NONE',  ( -0.000000000000000000, -0.000000000000000000, -1.000000000000000000 ) ) ;
#3358=DIRECTION ( 'NONE',  ( -0.000000000000000000, -0.000000000000000000, -1.000000000000000000 ) ) ;
#3360=DIRECTION ( 'NONE',  ( 0.000000000000000000, 0.000000000000000000, 1.000000000000000000 ) ) ;
#3363=ORIENTED_EDGE ( 'NONE', *, *, #2520, .F. ) ;
#3365=CARTESIAN_POINT ( 'NONE',  ( 74.61196207728339402, 28.86269417393366865, 38.99999999999995737 ) ) ;
#3366=DIRECTION ( 'NONE',  ( -0.3607836771741531612, -0.9326495259660494419, 0.000000000000000000 ) ) ;
#3371=ORIENTED_EDGE ( 'NONE', *, *, #2665, .T. ) ;
#3374=DIRECTION ( 'NONE',  ( -0.000000000000000000, -0.000000000000000000, 1.000000000000000000 ) ) ;
#3375=ORIENTED_EDGE ( 'NONE', *, *, #4636, .T. ) ;
#3376=DIRECTION ( 'NONE',  ( 0.000000000000000000, 0.000000000000000000, 1.000000000000000000 ) ) ;
#3380=EDGE_CURVE ( 'NONE', #2060, #3100, #484, .T. ) ;
#3382=CARTESIAN_POINT ( 'NONE',  ( 56.10121673609931037, 46.04269404270225863, 35.00000000000000000 ) ) ;
#3383=EDGE_LOOP ( 'NONE', ( #5739, #295 ) ) ;
#3386=ORIENTED_EDGE ( 'NONE', *, *, #5948, .F. ) ;
#3388=FACE_BOUND ( 'NONE', #1271, .T. ) ;
#3391=ORIENTED_EDGE ( 'NONE', *, *, #5841, .T. ) ;
#3393=ORIENTED_EDGE ( 'NONE', *, *, #5560, .F. ) ;
#3394=PLANE ( 'NONE',  #2167 ) ;
#3395=LINE ( 'NONE', #987, #2637 ) ;
#3403=EDGE_LOOP ( 'NONE', ( #290, #1507, #4130, #3893, #111 ) ) ;
#3404=FACE_OUTER_BOUND ( 'NONE', #5955, .T. ) ;
#3406=ORIENTED_EDGE ( 'NONE', *, *, #596, .T. ) ;
#3407=EDGE_CURVE ( 'NONE', #3100, #4900, #1888, .T. ) ;
#3409=LINE ( 'NONE', #935, #3748 ) ;
#3410=CARTESIAN_POINT ( 'NONE',  ( 0.000000000000000000, 0.000000000000000000, 38.99999999999995737 ) ) ;
#3413=DIRECTION ( 'NONE',  ( 1.000000000000000000, 0.000000000000000000, 0.000000000000000000 ) ) ;
#3414=EDGE_CURVE ( 'NONE', #816, #1974, #3783, .T. ) ;
#3416=CARTESIAN_POINT ( 'NONE',  ( 12.00215801354769063, 70.99259259259262933, 35.00000000000000000 ) ) ;
#3417=EDGE_LOOP ( 'NONE', ( #78, #1738, #3769, #1957 ) ) ;
#3418=CARTESIAN_POINT ( 'NONE',  ( -12.31015466235523981, 79.04720167209522685, 38.99999999999995737 ) ) ;
#3420=ORIENTED_EDGE ( 'NONE', *, *, #2807, .T. ) ;
#3422=CIRCLE ( 'NONE', #2635, 4.999999999999997335 ) ;
#3425=DIRECTION ( 'NONE',  ( -0.7787725926866162496, 0.6273063437270229858, 0.000000000000000000 ) ) ;
#3427=EDGE_CURVE ( 'NONE', #3444, #429, #6060, .T. ) ;
#3429=DIRECTION ( 'NONE',  ( 1.000000000000000000, 0.000000000000000000, 0.000000000000000000 ) ) ;
#3430=ORIENTED_EDGE ( 'NONE', *, *, #4059, .T. ) ;
#3431=AXIS2_PLACEMENT_3D ( 'NONE', #2621, #3577, #1305 ) ;
#3433=EDGE_LOOP ( 'NONE', ( #851, #1824, #2358, #3737, #2676, #3757, #5003, #2283, #316, #5440 ) ) ;
#3436=DIRECTION ( 'NONE',  ( -0.000000000000000000, 0.000000000000000000, 1.000000000000000000 ) ) ;
#3437=AXIS2_PLACEMENT_3D ( 'NONE', #3195, #2583, #967 ) ;
#3438=CIRCLE ( 'NONE', #4216, 80.00000000000002842 ) ;
#3439=EDGE_CURVE ( 'NONE', #5370, #1998, #5760, .T. ) ;
#3440=ORIENTED_EDGE ( 'NONE', *, *, #818, .F. ) ;
#3441=LINE ( 'NONE', #2847, #1937 ) ;
#3444=VERTEX_POINT ( 'NONE', #4318 ) ;
#3448=CARTESIAN_POINT ( 'NONE',  ( 5.114554293134526134E-14, 6.349488965209711204E-14, -35.00000000000000000 ) ) ;
#3452=DIRECTION ( 'NONE',  ( -0.000000000000000000, -0.000000000000000000, -1.000000000000000000 ) ) ;
#3455=EDGE_CURVE ( 'NONE', #404, #1987, #72, .T. ) ;
#3456=ORIENTED_EDGE ( 'NONE', *, *, #1972, .T. ) ;
#3457=ORIENTED_EDGE ( 'NONE', *, *, #742, .T. ) ;
#3460=AXIS2_PLACEMENT_3D ( 'NONE', #2954, #1516, #3413 ) ;
#3462=DIRECTION ( 'NONE',  ( -0.000000000000000000, -0.000000000000000000, -1.000000000000000000 ) ) ;
#3463=CONICAL_SURFACE ( 'NONE', #4652, 80.00000000000000000, 0.7853981633974482790 ) ;
#3464=AXIS2_PLACEMENT_3D ( 'NONE', #4876, #1195, #2081 ) ;
#3465=ADVANCED_FACE ( 'NONE', ( #5770, #1492, #2329, #6135, #3388, #1858, #5301, #1043, #2919, #5456, #4924, #2989 ), #4985, .T. ) ;
#3466=VERTEX_POINT ( 'NONE', #3418 ) ;
#3469=CARTESIAN_POINT ( 'NONE',  ( -6.247143215332724651E-13, -89.46264649666795776, 40.00000000000000000 ) ) ;
#3470=VERTEX_POINT ( 'NONE', #732 ) ;
#3471=DIRECTION ( 'NONE',  ( 1.000000000000000000, 0.000000000000000000, 0.000000000000000000 ) ) ;
#3472=CIRCLE ( 'NONE', #4769, 80.00000000000000000 ) ;
#3479=ORIENTED_EDGE ( 'NONE', *, *, #3194, .F. ) ;
#3480=DIRECTION ( 'NONE',  ( 0.000000000000000000, 0.000000000000000000, 1.000000000000000000 ) ) ;
#3484=CARTESIAN_POINT ( 'NONE',  ( 67.48246767247772482, 25.10212255632982092, 35.00000000000000000 ) ) ;
#3485=ORIENTED_EDGE ( 'NONE', *, *, #4457, .T. ) ;
#3486=DIRECTION ( 'NONE',  ( -0.5000000000000039968, 0.8660254037844363761, 0.000000000000000000 ) ) ;
#3487=PLANE ( 'NONE',  #1187 ) ;
#3488=CARTESIAN_POINT ( 'NONE',  ( 57.58482424179591419, -72.37680137756305498, 40.00000000000000000 ) ) ;
#3490=ORIENTED_EDGE ( 'NONE', *, *, #4954, .F. ) ;
#3494=EDGE_CURVE ( 'NONE', #2051, #3675, #4387, .T. ) ;
#3495=ORIENTED_EDGE ( 'NONE', *, *, #3343, .T. ) ;
#3496=DIRECTION ( 'NONE',  ( 0.9880900209011910240, -0.1538769332794358846, 0.000000000000000000 ) ) ;
#3499=FACE_BOUND ( 'NONE', #3767, .T. ) ;
#3502=LINE ( 'NONE', #5306, #1823 ) ;
#3503=ORIENTED_EDGE ( 'NONE', *, *, #1200, .F. ) ;
#3505=DIRECTION ( 'NONE',  ( -0.000000000000000000, 0.000000000000000000, 1.000000000000000000 ) ) ;
#3507=EDGE_LOOP ( 'NONE', ( #5769, #3230, #5311, #139 ) ) ;
#3509=ORIENTED_EDGE ( 'NONE', *, *, #1519, .T. ) ;
#3513=CARTESIAN_POINT ( 'NONE',  ( 5.000000000000003553, 89.46264649666795776, -79.99999999999998579 ) ) ;
#3514=FACE_OUTER_BOUND ( 'NONE', #4102, .T. ) ;
#3521=VECTOR ( 'NONE', #5584, 1000.000000000000000 ) ;
#3522=VECTOR ( 'NONE', #5768, 1000.000000000000000 ) ;
#3523=VERTEX_POINT ( 'NONE', #166 ) ;
#3524=CARTESIAN_POINT ( 'NONE',  ( 0.000000000000000000, 0.000000000000000000, -40.00000000000000000 ) ) ;
#3529=EDGE_CURVE ( 'NONE', #5996, #3051, #5967, .T. ) ;
#3530=CARTESIAN_POINT ( 'NONE',  ( -80.00000000000000000, 9.797174393178826052E-15, 38.99999999999995737 ) ) ;
#3531=CIRCLE ( 'NONE', #2547, 12.50000000000138733 ) ;
#3533=CIRCLE ( 'NONE', #2450, 5.000000000000004441 ) ;
#3535=EDGE_CURVE ( 'NONE', #1135, #4471, #3472, .T. ) ;
#3537=CARTESIAN_POINT ( 'NONE',  ( -85.08403291566612836, -27.64547812922793923, -40.00000000000000000 ) ) ;
#3539=FACE_OUTER_BOUND ( 'NONE', #4610, .T. ) ;
#3540=LINE ( 'NONE', #3911, #212 ) ;
#3542=EDGE_CURVE ( 'NONE', #4405, #5737, #3540, .T. ) ;
#3543=ORIENTED_EDGE ( 'NONE', *, *, #366, .F. ) ;
#3546=FACE_OUTER_BOUND ( 'NONE', #1911, .T. ) ;
#3549=LINE ( 'NONE', #1169, #4879 ) ;
#3551=ORIENTED_EDGE ( 'NONE', *, *, #1593, .F. ) ;
#3554=DIRECTION ( 'NONE',  ( 0.8660254037844385966, -0.5000000000000001110, 0.000000000000000000 ) ) ;
#3556=DIRECTION ( 'NONE',  ( -0.000000000000000000, 0.000000000000000000, 1.000000000000000000 ) ) ;
#3558=AXIS2_PLACEMENT_3D ( 'NONE', #2899, #4801, #1864 ) ;
#3560=EDGE_LOOP ( 'NONE', ( #3970, #3391, #5664, #2786, #4475, #3814, #5198 ) ) ;
#3561=FACE_BOUND ( 'NONE', #4799, .T. ) ;
#3562=VECTOR ( 'NONE', #4510, 1000.000000000000000 ) ;
#3565=DIRECTION ( 'NONE',  ( -0.000000000000000000, -0.000000000000000000, 1.000000000000000000 ) ) ;
#3566=VERTEX_POINT ( 'NONE', #5366 ) ;
#3571=CARTESIAN_POINT ( 'NONE',  ( 68.32682326288126262, 26.05379589900813997, 35.04915833130704073 ) ) ;
#3572=ORIENTED_EDGE ( 'NONE', *, *, #5455, .F. ) ;
#3574=CARTESIAN_POINT ( 'NONE',  ( 7.182140071210238271E-14, -8.916303653273167033E-14, 35.00000000000000000 ) ) ;
#3576=EDGE_CURVE ( 'NONE', #2489, #3996, #309, .T. ) ;
#3577=DIRECTION ( 'NONE',  ( 0.5000000000000001110, 0.8660254037844385966, -0.000000000000000000 ) ) ;
#3578=EDGE_CURVE ( 'NONE', #4471, #2132, #2838, .T. ) ;
#3580=CARTESIAN_POINT ( 'NONE',  ( -80.08403291566614257, -27.64547812922793923, 40.00000000000000000 ) ) ;
#3583=DIRECTION ( 'NONE',  ( -0.000000000000000000, 0.000000000000000000, 1.000000000000000000 ) ) ;
#3584=DIRECTION ( 'NONE',  ( 0.000000000000000000, 0.000000000000000000, 1.000000000000000000 ) ) ;
#3586=DIRECTION ( 'NONE',  ( -0.000000000000000000, -0.000000000000000000, -1.000000000000000000 ) ) ;
#3588=ORIENTED_EDGE ( 'NONE', *, *, #641, .T. ) ;
#3589=CARTESIAN_POINT ( 'NONE',  ( 4.130675435985391572E-14, 1.067806758184284836E-13, 35.00000000000000000 ) ) ;
#3596=VERTEX_POINT ( 'NONE', #1052 ) ;
#3598=EDGE_LOOP ( 'NONE', ( #644, #1428, #5177, #394, #1856, #3117 ) ) ;
#3599=CARTESIAN_POINT ( 'NONE',  ( -58.45671475544968843, 33.74999999999987210, 35.00000000000000000 ) ) ;
#3600=EDGE_CURVE ( 'NONE', #193, #537, #4742, .T. ) ;
#3603=DIRECTION ( 'NONE',  ( 0.6273063437270283149, 0.7787725926866119197, -0.000000000000000000 ) ) ;
#3604=DIRECTION ( 'NONE',  ( 1.000000000000000000, 0.000000000000000000, 0.000000000000000000 ) ) ;
#3605=ORIENTED_EDGE ( 'NONE', *, *, #3910, .F. ) ;
#3606=CARTESIAN_POINT ( 'NONE',  ( -12.00215801354939948, 70.99259259259233090, 35.00000000000000000 ) ) ;
#3614=ORIENTED_EDGE ( 'NONE', *, *, #1663, .T. ) ;
#3615=EDGE_CURVE ( 'NONE', #4405, #1185, #3171, .T. ) ;
#3616=FACE_BOUND ( 'NONE', #1491, .T. ) ;
#3618=AXIS2_PLACEMENT_3D ( 'NONE', #4023, #4949, #4111 ) ;
#3620=LINE ( 'NONE', #4532, #5236 ) ;
#3621=CIRCLE ( 'NONE', #6027, 72.00000000000004263 ) ;
#3622=FACE_OUTER_BOUND ( 'NONE', #4515, .T. ) ;
#3624=AXIS2_PLACEMENT_3D ( 'NONE', #5685, #1290, #503 ) ;
#3625=CIRCLE ( 'NONE', #165, 5.000000000000005329 ) ;
#3627=CIRCLE ( 'NONE', #2138, 9.999999999999996447 ) ;
#3628=ORIENTED_EDGE ( 'NONE', *, *, #1483, .F. ) ;
#3630=ORIENTED_EDGE ( 'NONE', *, *, #4636, .F. ) ;
#3631=CARTESIAN_POINT ( 'NONE',  ( -1.630640067418198669E-13, 67.50000000000002842, 35.00000000000000000 ) ) ;
#3632=AXIS2_PLACEMENT_3D ( 'NONE', #1716, #378, #1319 ) ;
#3635=DIRECTION ( 'NONE',  ( -0.000000000000000000, -0.000000000000000000, -1.000000000000000000 ) ) ;
#3636=CARTESIAN_POINT ( 'NONE',  ( -100.0000000000000000, 0.000000000000000000, 39.00000000000007105 ) ) ;
#3638=ADVANCED_FACE ( 'NONE', ( #1469 ), #2474, .F. ) ;
#3642=LINE ( 'NONE', #3183, #5719 ) ;
#3648=EDGE_LOOP ( 'NONE', ( #4069, #1163, #6007, #3273 ) ) ;
#3650=CARTESIAN_POINT ( 'NONE',  ( 52.58482424179643289, 72.37680137756268550, 40.00000000000000000 ) ) ;
#3651=AXIS2_PLACEMENT_3D ( 'NONE', #4293, #5207, #44 ) ;
#3652=PLANE ( 'NONE',  #4434 ) ;
#3654=AXIS2_PLACEMENT_3D ( 'NONE', #439, #2319, #6039 ) ;
#3655=CARTESIAN_POINT ( 'NONE',  ( -9.192833548570215285, -59.02994620157096506, 35.00000000000000000 ) ) ;
#3656=DIRECTION ( 'NONE',  ( -0.1538769332794488742, 0.9880900209011889146, 0.000000000000000000 ) ) ;
#3657=AXIS2_PLACEMENT_3D ( 'NONE', #268, #3058, #629 ) ;
#3658=AXIS2_PLACEMENT_3D ( 'NONE', #4297, #496, #2409 ) ;
#3659=DIRECTION ( 'NONE',  ( 1.000000000000000000, 0.000000000000000000, 0.000000000000000000 ) ) ;
#3660=VERTEX_POINT ( 'NONE', #2902 ) ;
#3661=CARTESIAN_POINT ( 'NONE',  ( 0.000000000000000000, 0.000000000000000000, 40.00000000000000000 ) ) ;
#3662=ORIENTED_EDGE ( 'NONE', *, *, #2064, .T. ) ;
#3663=CYLINDRICAL_SURFACE ( 'NONE', #1966, 12.50000000000000355 ) ;
#3664=CARTESIAN_POINT ( 'NONE',  ( 46.52501622030442974, -37.47620048660870395, 35.00000000000000000 ) ) ;
#3665=PLANE ( 'NONE',  #2036 ) ;
#3666=PLANE ( 'NONE',  #1771 ) ;
#3669=EDGE_LOOP ( 'NONE', ( #4359, #1638, #5172, #1217 ) ) ;
#3670=DIRECTION ( 'NONE',  ( -0.9326495259660518844, 0.3607836771741464998, 0.000000000000000000 ) ) ;
#3671=DIRECTION ( 'NONE',  ( -0.4999999999999920619, -0.8660254037844432595, 0.000000000000000000 ) ) ;
#3672=LINE ( 'NONE', #3277, #86 ) ;
#3675=VERTEX_POINT ( 'NONE', #1830 ) ;
#3677=CARTESIAN_POINT ( 'NONE',  ( -54.99999999999990052, -21.27605460800010206, -35.00000000000000000 ) ) ;
#3678=ADVANCED_FACE ( 'NONE', ( #990 ), #1004, .F. ) ;
#3679=EDGE_CURVE ( 'NONE', #2846, #3566, #3730, .T. ) ;
#3681=CARTESIAN_POINT ( 'NONE',  ( -99.00000000000005684, 0.000000000000000000, 40.00000000000000000 ) ) ;
#3683=ADVANCED_FACE ( 'NONE', ( #5182 ), #3755, .F. ) ;
#3686=ORIENTED_EDGE ( 'NONE', *, *, #2015, .T. ) ;
#3687=FACE_OUTER_BOUND ( 'NONE', #5877, .T. ) ;
#3688=ORIENTED_EDGE ( 'NONE', *, *, #1857, .F. ) ;
#3694=DIRECTION ( 'NONE',  ( 0.000000000000000000, 0.000000000000000000, 1.000000000000000000 ) ) ;
#3697=FACE_OUTER_BOUND ( 'NONE', #2765, .T. ) ;
#3700=CARTESIAN_POINT ( 'NONE',  ( -57.35713647667095927, -46.20154318182582642, 35.13717928826310555 ) ) ;
#3703=FACE_OUTER_BOUND ( 'NONE', #5011, .T. ) ;
#3705=DIRECTION ( 'NONE',  ( -0.5000000000000037748, 0.8660254037844365982, 0.000000000000000000 ) ) ;
#3715=DIRECTION ( 'NONE',  ( 1.000000000000000000, 0.000000000000000000, 0.000000000000000000 ) ) ;
#3716=DIRECTION ( 'NONE',  ( 0.000000000000000000, 0.000000000000000000, 1.000000000000000000 ) ) ;
#3717=CARTESIAN_POINT ( 'NONE',  ( 80.00000000000000000, 0.000000000000000000, 38.99999999999995737 ) ) ;
#3718=ORIENTED_EDGE ( 'NONE', *, *, #2168, .T. ) ;
#3719=DIRECTION ( 'NONE',  ( 0.1538769332794359124, 0.9880900209011910240, 0.000000000000000000 ) ) ;
#3720=CIRCLE ( 'NONE', #179, 80.00000000000000000 ) ;
#3721=ADVANCED_FACE ( 'NONE', ( #3335 ), #5249, .F. ) ;
#3724=ORIENTED_EDGE ( 'NONE', *, *, #2168, .F. ) ;
#3725=CARTESIAN_POINT ( 'NONE',  ( 55.71784976887228424, -21.55374571496028224, 35.00000000000000000 ) ) ;
#3726=DIRECTION ( 'NONE',  ( 0.4999999999999980016, 0.8660254037844398178, 0.000000000000000000 ) ) ;
#3730=LINE ( 'NONE', #1374, #403 ) ;
#3734=VERTEX_POINT ( 'NONE', #3983 ) ;
#3736=PLANE ( 'NONE',  #3624 ) ;
#3737=ORIENTED_EDGE ( 'NONE', *, *, #4145, .F. ) ;
#3738=CARTESIAN_POINT ( 'NONE',  ( 0.000000000000000000, 0.000000000000000000, -35.00000000000000000 ) ) ;
#3740=CARTESIAN_POINT ( 'NONE',  ( -74.61196207728360719, -28.86269417393315351, -35.00000000000000711 ) ) ;
#3741=VECTOR ( 'NONE', #4578, 1000.000000000000000 ) ;
#3742=DIRECTION ( 'NONE',  ( 0.1538769332794487910, -0.9880900209011889146, 0.000000000000000000 ) ) ;
#3743=AXIS2_PLACEMENT_3D ( 'NONE', #3661, #6008, #1722 ) ;
#3744=CIRCLE ( 'NONE', #4755, 4.999999999999990230 ) ;
#3747=DIRECTION ( 'NONE',  ( -0.000000000000000000, 0.000000000000000000, 1.000000000000000000 ) ) ;
#3748=VECTOR ( 'NONE', #4788, 1000.000000000000000 ) ;
#3750=CARTESIAN_POINT ( 'NONE',  ( -85.08403291566554572, 27.64547812922971914, 40.00000000000000000 ) ) ;
#3752=EDGE_CURVE ( 'NONE', #2272, #5491, #5900, .T. ) ;
#3754=ORIENTED_EDGE ( 'NONE', *, *, #5560, .T. ) ;
#3755=TOROIDAL_SURFACE ( 'NONE', #2, 72.00000000000004263, 10.00000000000000000 ) ;
#3757=ORIENTED_EDGE ( 'NONE', *, *, #1603, .F. ) ;
#3758=ORIENTED_EDGE ( 'NONE', *, *, #1603, .T. ) ;
#3759=DIRECTION ( 'NONE',  ( 1.000000000000000000, 0.000000000000000000, 0.000000000000000000 ) ) ;
#3761=EDGE_CURVE ( 'NONE', #1713, #2020, #4365, .T. ) ;
#3762=CARTESIAN_POINT ( 'NONE',  ( 100.0000000000000000, 1.224646799147353217E-14, 40.00000000000000000 ) ) ;
#3763=DIRECTION ( 'NONE',  ( 0.000000000000000000, 0.000000000000000000, 1.000000000000000000 ) ) ;
#3764=ADVANCED_FACE ( 'NONE', ( #1996 ), #5374, .F. ) ;
#3766=DIRECTION ( 'NONE',  ( -1.000000000000000000, 0.000000000000000000, 0.000000000000000000 ) ) ;
#3767=EDGE_LOOP ( 'NONE', ( #3879, #1876 ) ) ;
#3769=ORIENTED_EDGE ( 'NONE', *, *, #3921, .F. ) ;
#3770=DIRECTION ( 'NONE',  ( -0.1538769332794359124, -0.9880900209011910240, 0.000000000000000000 ) ) ;
#3772=PLANE ( 'NONE',  #2236 ) ;
#3776=CARTESIAN_POINT ( 'NONE',  ( 12.31015466235495026, 79.04720167209526949, 38.99999999999995737 ) ) ;
#3778=ORIENTED_EDGE ( 'NONE', *, *, #2813, .F. ) ;
#3779=DIRECTION ( 'NONE',  ( -0.000000000000000000, -0.000000000000000000, 1.000000000000000000 ) ) ;
#3780=CARTESIAN_POINT ( 'NONE',  ( 9.192833548570416013, -59.02994620156847105, 35.00000000000000000 ) ) ;
#3781=FACE_OUTER_BOUND ( 'NONE', #1095, .T. ) ;
#3783=LINE ( 'NONE', #5203, #2581 ) ;
#3787=EDGE_LOOP ( 'NONE', ( #4452, #171, #477, #567 ) ) ;
#3788=VERTEX_POINT ( 'NONE', #1615 ) ;
#3789=CARTESIAN_POINT ( 'NONE',  ( 81.00000000000004263, 0.000000000000000000, 40.00000000000000000 ) ) ;
#3791=DIRECTION ( 'NONE',  ( -0.9326495259660445569, -0.3607836771741652071, 0.000000000000000000 ) ) ;
#3800=VERTEX_POINT ( 'NONE', #740 ) ;
#3801=CARTESIAN_POINT ( 'NONE',  ( -58.45671475544962448, -33.75000000000001421, 35.00000000000000000 ) ) ;
#3802=ADVANCED_FACE ( 'NONE', ( #5401 ), #1141, .F. ) ;
#3804=DIRECTION ( 'NONE',  ( -0.000000000000000000, -0.000000000000000000, -1.000000000000000000 ) ) ;
#3809=CARTESIAN_POINT ( 'NONE',  ( 47.58482424179590708, -72.37680137756305498, -79.99999999999998579 ) ) ;
#3810=CARTESIAN_POINT ( 'NONE',  ( 0.000000000000000000, 0.000000000000000000, 40.00000000000000000 ) ) ;
#3811=AXIS2_PLACEMENT_3D ( 'NONE', #4701, #1370, #3671 ) ;
#3812=AXIS2_PLACEMENT_3D ( 'NONE', #1953, #914, #1914 ) ;
#3813=CARTESIAN_POINT ( 'NONE',  ( 0.000000000000000000, 67.50000000000000000, 35.00000000000000000 ) ) ;
#3814=ORIENTED_EDGE ( 'NONE', *, *, #2448, .T. ) ;
#3815=CARTESIAN_POINT ( 'NONE',  ( -85.08403291566554572, 27.64547812922971914, -40.00000000000000000 ) ) ;
#3818=CIRCLE ( 'NONE', #1734, 12.50000000000138733 ) ;
#3822=CARTESIAN_POINT ( 'NONE',  ( 0.000000000000000000, 0.000000000000000000, 38.99999999999995737 ) ) ;
#3824=CIRCLE ( 'NONE', #471, 5.000000000000004441 ) ;
#3825=CARTESIAN_POINT ( 'NONE',  ( 0.000000000000000000, 0.000000000000000000, 45.00000000000000711 ) ) ;
#3828=CIRCLE ( 'NONE', #4629, 5.000000000000004441 ) ;
#3830=ORIENTED_EDGE ( 'NONE', *, *, #2636, .F. ) ;
#3832=CARTESIAN_POINT ( 'NONE',  ( 67.48246767247772482, 25.10212255632982092, 35.00000000000000000 ) ) ;
#3833=CARTESIAN_POINT ( 'NONE',  ( 0.000000000000000000, 0.000000000000000000, -39.00000000000002842 ) ) ;
#3835=EDGE_CURVE ( 'NONE', #4044, #3444, #213, .T. ) ;
#3836=VERTEX_POINT ( 'NONE', #3891 ) ;
#3837=CARTESIAN_POINT ( 'NONE',  ( 0.000000000000000000, 0.000000000000000000, -35.00000000000000000 ) ) ;
#3841=EDGE_CURVE ( 'NONE', #5491, #537, #3549, .T. ) ;
#3842=DIRECTION ( 'NONE',  ( -0.000000000000000000, 0.000000000000000000, 1.000000000000000000 ) ) ;
#3844=CARTESIAN_POINT ( 'NONE',  ( -12.49999999999999822, -67.50000000000000000, 35.00000000000000000 ) ) ;
#3848=CIRCLE ( 'NONE', #1269, 12.50000000000138911 ) ;
#3850=ORIENTED_EDGE ( 'NONE', *, *, #1333, .T. ) ;
#3851=CARTESIAN_POINT ( 'NONE',  ( 4.130675435985391572E-14, 1.067806758184284836E-13, 35.00000000000000000 ) ) ;
#3852=VECTOR ( 'NONE', #2455, 1000.000000000000114 ) ;
#3854=ORIENTED_EDGE ( 'NONE', *, *, #3236, .T. ) ;
#3856=VERTEX_POINT ( 'NONE', #4425 ) ;
#3857=AXIS2_PLACEMENT_3D ( 'NONE', #738, #177, #1589 ) ;
#3859=LINE ( 'NONE', #2433, #3131 ) ;
#3865=VERTEX_POINT ( 'NONE', #3488 ) ;
#3867=DIRECTION ( 'NONE',  ( 0.000000000000000000, 0.000000000000000000, 1.000000000000000000 ) ) ;
#3868=CARTESIAN_POINT ( 'NONE',  ( -56.10121673609931037, -46.04269404270225863, 35.00000000000000000 ) ) ;
#3869=ORIENTED_EDGE ( 'NONE', *, *, #2697, .T. ) ;
#3870=DIRECTION ( 'NONE',  ( -0.8660254037844385966, 0.5000000000000001110, 0.000000000000000000 ) ) ;
#3872=ORIENTED_EDGE ( 'NONE', *, *, #2318, .F. ) ;
#3873=EDGE_CURVE ( 'NONE', #559, #5737, #5426, .T. ) ;
#3874=EDGE_CURVE ( 'NONE', #2223, #719, #3022, .T. ) ;
#3875=CARTESIAN_POINT ( 'NONE',  ( 67.48246767247886169, -25.10212255632678691, 35.00000000000000000 ) ) ;
#3876=CARTESIAN_POINT ( 'NONE',  ( 11.33314185116896589, 72.77350886803867525, 35.00000000000000000 ) ) ;
#3877=ADVANCED_FACE ( 'NONE', ( #685 ), #1929, .F. ) ;
#3878=CARTESIAN_POINT ( 'NONE',  ( 57.35713647667095927, 46.20154318182582642, 35.13717928826310555 ) ) ;
#3879=ORIENTED_EDGE ( 'NONE', *, *, #4598, .T. ) ;
#3880=DIRECTION ( 'NONE',  ( -0.000000000000000000, -0.000000000000000000, 1.000000000000000000 ) ) ;
#3881=CARTESIAN_POINT ( 'NONE',  ( 54.99999999999999289, 6.349087922075113966E-13, 35.00000000000000000 ) ) ;
#3883=ORIENTED_EDGE ( 'NONE', *, *, #1663, .F. ) ;
#3885=EDGE_CURVE ( 'NONE', #6127, #2468, #2566, .T. ) ;
#3886=VERTEX_POINT ( 'NONE', #4965 ) ;
#3888=DIRECTION ( 'NONE',  ( 0.000000000000000000, 0.000000000000000000, 1.000000000000000000 ) ) ;
#3891=CARTESIAN_POINT ( 'NONE',  ( -57.35713647667095927, -46.20154318182582642, -35.00000000000000000 ) ) ;
#3893=ORIENTED_EDGE ( 'NONE', *, *, #4270, .T. ) ;
#3894=ORIENTED_EDGE ( 'NONE', *, *, #5266, .T. ) ;
#3897=CARTESIAN_POINT ( 'NONE',  ( 0.000000000000000000, 0.000000000000000000, 35.00000000000000000 ) ) ;
#3898=ORIENTED_EDGE ( 'NONE', *, *, #5521, .F. ) ;
#3903=EDGE_CURVE ( 'NONE', #4711, #5893, #162, .T. ) ;
#3906=VERTEX_POINT ( 'NONE', #1769 ) ;
#3907=CARTESIAN_POINT ( 'NONE',  ( 85.08403291566592941, 27.64547812922851833, 40.00000000000000000 ) ) ;
#3908=CARTESIAN_POINT ( 'NONE',  ( 1.131281550719567528E-13, 1.761763928569687004E-14, 35.00000000000000000 ) ) ;
#3909=DIRECTION ( 'NONE',  ( 0.000000000000000000, 0.000000000000000000, 1.000000000000000000 ) ) ;
#3910=EDGE_CURVE ( 'NONE', #719, #2891, #463, .T. ) ;
#3911=CARTESIAN_POINT ( 'NONE',  ( 68.69027832783777399, 26.57196568621521138, 35.00000000000000000 ) ) ;
#3913=ORIENTED_EDGE ( 'NONE', *, *, #3003, .F. ) ;
#3915=VECTOR ( 'NONE', #2714, 1000.000000000000000 ) ;
#3916=ORIENTED_EDGE ( 'NONE', *, *, #5377, .T. ) ;
#3920=DIRECTION ( 'NONE',  ( -0.000000000000000000, -0.000000000000000000, -1.000000000000000000 ) ) ;
#3921=EDGE_CURVE ( 'NONE', #747, #5424, #332, .T. ) ;
#3922=LINE ( 'NONE', #5844, #2172 ) ;
#3923=VECTOR ( 'NONE', #823, 999.9999999999998863 ) ;
#3924=VECTOR ( 'NONE', #6133, 1000.000000000000114 ) ;
#3927=DIRECTION ( 'NONE',  ( 0.9326495259660518844, -0.3607836771741464998, 0.000000000000000000 ) ) ;
#3929=CIRCLE ( 'NONE', #5722, 10.00000000000000178 ) ;
#3930=AXIS2_PLACEMENT_3D ( 'NONE', #2667, #5393, #2956 ) ;
#3931=EDGE_LOOP ( 'NONE', ( #1112, #3628, #3108, #5556, #5232 ) ) ;
#3933=AXIS2_PLACEMENT_3D ( 'NONE', #4850, #1029, #601 ) ;
#3935=ORIENTED_EDGE ( 'NONE', *, *, #4999, .F. ) ;
#3936=VECTOR ( 'NONE', #3880, 1000.000000000000000 ) ;
#3939=CIRCLE ( 'NONE', #189, 12.50000000000138911 ) ;
#3941=CARTESIAN_POINT ( 'NONE',  ( 99.00000000000005684, 1.212400331155880333E-14, 40.00000000000000000 ) ) ;
#3942=ORIENTED_EDGE ( 'NONE', *, *, #5828, .F. ) ;
#3943=CARTESIAN_POINT ( 'NONE',  ( -85.08403291566612836, -27.64547812922793923, 40.00000000000000000 ) ) ;
#3947=EDGE_LOOP ( 'NONE', ( #5674, #1905, #1455, #1281 ) ) ;
#3950=DIRECTION ( 'NONE',  ( 0.4999999999999980016, 0.8660254037844398178, 0.000000000000000000 ) ) ;
#3952=ADVANCED_FACE ( 'NONE', ( #267 ), #358, .F. ) ;
#3953=CARTESIAN_POINT ( 'NONE',  ( -5.000000000000003553, 89.46264649666795776, 40.00000000000000000 ) ) ;
#3958=ORIENTED_EDGE ( 'NONE', *, *, #241, .T. ) ;
#3960=ORIENTED_EDGE ( 'NONE', *, *, #531, .F. ) ;
#3961=ADVANCED_FACE ( 'NONE', ( #1331 ), #3665, .F. ) ;
#3963=AXIS2_PLACEMENT_3D ( 'NONE', #2535, #4426, #2059 ) ;
#3964=LINE ( 'NONE', #5879, #4444 ) ;
#3965=CARTESIAN_POINT ( 'NONE',  ( 11.33314185117008677, -72.77350886804093477, 35.13717928826310555 ) ) ;
#3966=VERTEX_POINT ( 'NONE', #5579 ) ;
#3967=VECTOR ( 'NONE', #447, 1000.000000000000114 ) ;
#3970=ORIENTED_EDGE ( 'NONE', *, *, #1373, .F. ) ;
#3973=DIRECTION ( 'NONE',  ( -0.9326495259660493309, 0.3607836771741531612, 0.000000000000000000 ) ) ;
#3974=ORIENTED_EDGE ( 'NONE', *, *, #723, .F. ) ;
#3975=CARTESIAN_POINT ( 'NONE',  ( 80.08403291566574467, -27.64547812922912939, -79.99999999999998579 ) ) ;
#3978=CARTESIAN_POINT ( 'NONE',  ( 74.61196207728411878, -28.86269417393183190, 38.99999999999995737 ) ) ;
#3979=EDGE_LOOP ( 'NONE', ( #5870, #2684, #919, #5351 ) ) ;
#3980=CARTESIAN_POINT ( 'NONE',  ( -5.114554293134481958E-14, -6.349488965209747807E-14, -35.00000000000000000 ) ) ;
#3981=FACE_OUTER_BOUND ( 'NONE', #5169, .T. ) ;
#3983=CARTESIAN_POINT ( 'NONE',  ( -72.00000000000004263, 0.000000000000000000, 35.00000000000000000 ) ) ;
#3985=ORIENTED_EDGE ( 'NONE', *, *, #2230, .T. ) ;
#3986=ADVANCED_FACE ( 'NONE', ( #3235 ), #4099, .F. ) ;
#3987=ADVANCED_FACE ( 'NONE', ( #1795 ), #6118, .F. ) ;
#3988=ORIENTED_EDGE ( 'NONE', *, *, #5073, .F. ) ;
#3992=ORIENTED_EDGE ( 'NONE', *, *, #5502, .F. ) ;
#3994=EDGE_CURVE ( 'NONE', #5424, #816, #3145, .T. ) ;
#3996=VERTEX_POINT ( 'NONE', #5604 ) ;
#3997=CARTESIAN_POINT ( 'NONE',  ( 0.000000000000000000, -67.50000000000000000, 35.00000000000000000 ) ) ;
#4001=VERTEX_POINT ( 'NONE', #4547 ) ;
#4002=DIRECTION ( 'NONE',  ( -0.000000000000000000, -0.000000000000000000, 1.000000000000000000 ) ) ;
#4004=VERTEX_POINT ( 'NONE', #1678 ) ;
#4006=ORIENTED_EDGE ( 'NONE', *, *, #1869, .F. ) ;
#4007=DIRECTION ( 'NONE',  ( -0.7787725926866162496, 0.6273063437270229858, 0.000000000000000000 ) ) ;
#4009=PRODUCT_CONTEXT ( 'NONE', #2134, 'mechanical' ) ;
#4010=DIRECTION ( 'NONE',  ( 0.7787725926866080339, 0.6273063437270329779, 0.000000000000000000 ) ) ;
#4012=ORIENTED_EDGE ( 'NONE', *, *, #3198, .F. ) ;
#4016=AXIS2_PLACEMENT_3D ( 'NONE', #5915, #3103, #5010 ) ;
#4021=VECTOR ( 'NONE', #4826, 1000.000000000000000 ) ;
#4022=DIRECTION ( 'NONE',  ( -0.000000000000000000, -0.000000000000000000, 1.000000000000000000 ) ) ;
#4023=CARTESIAN_POINT ( 'NONE',  ( 85.08403291566575888, -27.64547812922912939, -40.00000000000000000 ) ) ;
#4025=AXIS2_PLACEMENT_3D ( 'NONE', #3027, #5436, #5030 ) ;
#4026=VECTOR ( 'NONE', #6066, 1000.000000000000000 ) ;
#4028=ADVANCED_FACE ( 'NONE', ( #2148 ), #2268, .F. ) ;
#4029=LINE ( 'NONE', #2100, #1539 ) ;
#4031=ORIENTED_EDGE ( 'NONE', *, *, #99, .T. ) ;
#4033=VECTOR ( 'NONE', #3219, 1000.000000000000000 ) ;
#4035=ORIENTED_EDGE ( 'NONE', *, *, #4210, .T. ) ;
#4036=DIRECTION ( 'NONE',  ( 0.000000000000000000, 0.000000000000000000, 1.000000000000000000 ) ) ;
#4037=VERTEX_POINT ( 'NONE', #5086 ) ;
#4038=DIRECTION ( 'NONE',  ( 0.000000000000000000, 0.000000000000000000, 1.000000000000000000 ) ) ;
#4039=CARTESIAN_POINT ( 'NONE',  ( -9.074396217167327805, 58.26942451214400620, -35.00000000000000000 ) ) ;
#4041=DIRECTION ( 'NONE',  ( 1.000000000000000000, 0.000000000000000000, 0.000000000000000000 ) ) ;
#4042=CARTESIAN_POINT ( 'NONE',  ( 9.074396217167167933, 58.26942451214404173, 35.00000000000000000 ) ) ;
#4043=CIRCLE ( 'NONE', #1180, 80.00000000000000000 ) ;
#4044=VERTEX_POINT ( 'NONE', #1224 ) ;
#4046=DIRECTION ( 'NONE',  ( -0.000000000000000000, -0.000000000000000000, -1.000000000000000000 ) ) ;
#4047=CYLINDRICAL_SURFACE ( 'NONE', #4839, 12.50000000000138556 ) ;
#4048=CIRCLE ( 'NONE', #4247, 100.0000000000000000 ) ;
#4049=ORIENTED_EDGE ( 'NONE', *, *, #3576, .T. ) ;
#4051=DIRECTION ( 'NONE',  ( 1.000000000000000000, 0.000000000000000000, 0.000000000000000000 ) ) ;
#4052=CIRCLE ( 'NONE', #2477, 12.49999999999999822 ) ;
#4054=CIRCLE ( 'NONE', #1279, 4.999999999999997335 ) ;
#4055=ORIENTED_EDGE ( 'NONE', *, *, #5309, .T. ) ;
#4057=CARTESIAN_POINT ( 'NONE',  ( 12.31015466235579225, -79.04720167209512738, 35.00000000000000000 ) ) ;
#4059=EDGE_CURVE ( 'NONE', #2065, #132, #5723, .T. ) ;
#4060=ADVANCED_FACE ( 'NONE', ( #2184 ), #4072, .F. ) ;
#4061=CARTESIAN_POINT ( 'NONE',  ( 46.52501622030217021, 37.47620048660763103, -35.00000000000000000 ) ) ;
#4062=DIRECTION ( 'NONE',  ( 0.9880900209011890256, 0.1538769332794488465, -0.000000000000000000 ) ) ;
#4065=ADVANCED_FACE ( 'NONE', ( #2398 ), #482, .F. ) ;
#4067=EDGE_LOOP ( 'NONE', ( #3850, #590, #173, #2333 ) ) ;
#4069=ORIENTED_EDGE ( 'NONE', *, *, #5850, .T. ) ;
#4070=CARTESIAN_POINT ( 'NONE',  ( -12.00215801354769063, -70.99259259259262933, 35.00000000000000000 ) ) ;
#4072=PLANE ( 'NONE',  #5616 ) ;
#4080=CARTESIAN_POINT ( 'NONE',  ( -47.58482424179536707, 72.37680137756343868, -40.00000000000000000 ) ) ;
#4082=ORIENTED_EDGE ( 'NONE', *, *, #2056, .F. ) ;
#4085=EDGE_LOOP ( 'NONE', ( #3339, #5136 ) ) ;
#4086=DIRECTION ( 'NONE',  ( -1.000000000000000000, 0.000000000000000000, 0.000000000000000000 ) ) ;
#4087=( NAMED_UNIT ( * ) PLANE_ANGLE_UNIT ( ) SI_UNIT ( $, .RADIAN. ) );
#4090=VERTEX_POINT ( 'NONE', #4729 ) ;
#4091=EDGE_CURVE ( 'NONE', #4790, #3470, #4620, .T. ) ;
#4093=ORIENTED_EDGE ( 'NONE', *, *, #438, .T. ) ;
#4095=ORIENTED_EDGE ( 'NONE', *, *, #4407, .T. ) ;
#4096=CARTESIAN_POINT ( 'NONE',  ( 2.941541598353386116E-14, -7.604078429494091299E-14, 35.00000000000000000 ) ) ;
#4098=EDGE_CURVE ( 'NONE', #2846, #5114, #70, .T. ) ;
#4099=PLANE ( 'NONE',  #3431 ) ;
#4101=DIRECTION ( 'NONE',  ( -0.000000000000000000, 0.000000000000000000, 1.000000000000000000 ) ) ;
#4102=EDGE_LOOP ( 'NONE', ( #931, #3018, #3662, #1462 ) ) ;
#4103=CARTESIAN_POINT ( 'NONE',  ( 67.15076586955576943, -25.97642475653856664, 45.00000000000000711 ) ) ;
#4104=DIRECTION ( 'NONE',  ( -0.000000000000000000, -0.000000000000000000, -1.000000000000000000 ) ) ;
#4106=ADVANCED_FACE ( 'NONE', ( #519 ), #2364, .F. ) ;
#4111=DIRECTION ( 'NONE',  ( 1.000000000000000000, 0.000000000000000000, 0.000000000000000000 ) ) ;
#4112=TOROIDAL_SURFACE ( 'NONE', #4016, 72.00000000000004263, 10.00000000000000000 ) ;
#4113=CYLINDRICAL_SURFACE ( 'NONE', #965, 4.999999999999990230 ) ;
#4114=AXIS2_PLACEMENT_3D ( 'NONE', #2580, #2162, #2664 ) ;
#4115=AXIS2_PLACEMENT_3D ( 'NONE', #3813, #36, #2423 ) ;
#4116=DIRECTION ( 'NONE',  ( -0.000000000000000000, 0.000000000000000000, 1.000000000000000000 ) ) ;
#4117=AXIS2_PLACEMENT_3D ( 'NONE', #3750, #2795, #3321 ) ;
#4118=DIRECTION ( 'NONE',  ( -0.1538769332794488187, 0.9880900209011889146, 0.000000000000000000 ) ) ;
#4121=CIRCLE ( 'NONE', #5129, 80.00000000000000000 ) ;
#4123=VECTOR ( 'NONE', #1549, 1000.000000000000000 ) ;
#4126=CARTESIAN_POINT ( 'NONE',  ( 0.000000000000000000, 0.000000000000000000, -40.00000000000000000 ) ) ;
#4129=CARTESIAN_POINT ( 'NONE',  ( 54.99999999999975131, 21.27605460800048576, 35.00000000000000000 ) ) ;
#4130=ORIENTED_EDGE ( 'NONE', *, *, #4793, .T. ) ;
#4131=DIRECTION ( 'NONE',  ( 1.000000000000000000, 0.000000000000000000, 0.000000000000000000 ) ) ;
#4132=VECTOR ( 'NONE', #3082, 1000.000000000000000 ) ;
#4136=DIRECTION ( 'NONE',  ( -0.000000000000000000, -0.000000000000000000, -1.000000000000000000 ) ) ;
#4137=EDGE_CURVE ( 'NONE', #506, #2123, #4668, .T. ) ;
#4138=EDGE_CURVE ( 'NONE', #1185, #2223, #1066, .T. ) ;
#4139=ORIENTED_EDGE ( 'NONE', *, *, #3170, .T. ) ;
#4140=CARTESIAN_POINT ( 'NONE',  ( -5.000000000000003553, 89.46264649666795776, -40.00000000000000000 ) ) ;
#4145=EDGE_CURVE ( 'NONE', #5444, #1288, #4187, .T. ) ;
#4147=ORIENTED_EDGE ( 'NONE', *, *, #3994, .F. ) ;
#4149=CARTESIAN_POINT ( 'NONE',  ( -12.31015466235495026, -79.04720167209526949, 38.99999999999995737 ) ) ;
#4150=CARTESIAN_POINT ( 'NONE',  ( 0.000000000000000000, 0.000000000000000000, 38.99999999999995737 ) ) ;
#4152=DIRECTION ( 'NONE',  ( 0.000000000000000000, 0.000000000000000000, 1.000000000000000000 ) ) ;
#4154=DIRECTION ( 'NONE',  ( -0.000000000000000000, -0.000000000000000000, -1.000000000000000000 ) ) ;
#4155=AXIS2_PLACEMENT_3D ( 'NONE', #2799, #5173, #4697 ) ;
#4157=ORIENTED_EDGE ( 'NONE', *, *, #1322, .T. ) ;
#4158=CARTESIAN_POINT ( 'NONE',  ( 11.33314185117008677, -72.77350886804093477, -35.00000000000000000 ) ) ;
#4160=DIRECTION ( 'NONE',  ( -1.000000000000000000, 0.000000000000000000, 0.000000000000000000 ) ) ;
#4161=CARTESIAN_POINT ( 'NONE',  ( 55.00000000000024158, -21.27605460799916770, -35.00000000000000000 ) ) ;
#4164=CARTESIAN_POINT ( 'NONE',  ( 0.000000000000000000, 0.000000000000000000, -35.00000000000000000 ) ) ;
#4165=ORIENTED_EDGE ( 'NONE', *, *, #4457, .F. ) ;
#4167=DIRECTION ( 'NONE',  ( -0.000000000000000000, 0.000000000000000000, 1.000000000000000000 ) ) ;
#4168=CARTESIAN_POINT ( 'NONE',  ( -55.71784976887214924, 21.55374571496067304, 35.00000000000000000 ) ) ;
#4169=ADVANCED_FACE ( 'NONE', ( #3781 ), #1394, .F. ) ;
#4174=CARTESIAN_POINT ( 'NONE',  ( 12.00215801354769063, 70.99259259259262933, 35.00000000000000000 ) ) ;
#4175=ADVANCED_FACE ( 'NONE', ( #1458 ), #5635, .F. ) ;
#4177=CARTESIAN_POINT ( 'NONE',  ( 0.000000000000000000, 0.000000000000000000, 35.00000000000000000 ) ) ;
#4178=PLANE ( 'NONE',  #3632 ) ;
#4179=DIRECTION ( 'NONE',  ( -0.7787725926866080339, -0.6273063437270329779, 0.000000000000000000 ) ) ;
#4185=DIRECTION ( 'NONE',  ( -0.000000000000000000, 0.000000000000000000, 1.000000000000000000 ) ) ;
#4186=CYLINDRICAL_SURFACE ( 'NONE', #2965, 12.50000000000138556 ) ;
#4187=LINE ( 'NONE', #3717, #3924 ) ;
#4188=EDGE_LOOP ( 'NONE', ( #4082, #3614, #2399, #257 ) ) ;
#4190=CARTESIAN_POINT ( 'NONE',  ( -80.00000000000000000, 0.000000000000000000, 40.00000000000000000 ) ) ;
#4192=CARTESIAN_POINT ( 'NONE',  ( -68.69027832784050247, 26.57196568621489163, 35.00000000000000000 ) ) ;
#4193=LINE ( 'NONE', #6108, #1927 ) ;
#4196=MANIFOLD_SOLID_BREP ( 'Fillet1', #2459 ) ;
#4197=DIRECTION ( 'NONE',  ( 0.000000000000000000, 0.000000000000000000, 1.000000000000000000 ) ) ;
#4198=ORIENTED_EDGE ( 'NONE', *, *, #1323, .F. ) ;
#4201=DIRECTION ( 'NONE',  ( 1.000000000000000000, 0.000000000000000000, 0.000000000000000000 ) ) ;
#4203=DIRECTION ( 'NONE',  ( 1.000000000000000000, 0.000000000000000000, 0.000000000000000000 ) ) ;
#4205=VECTOR ( 'NONE', #4552, 1000.000000000000000 ) ;
#4206=EDGE_CURVE ( 'NONE', #4976, #3788, #2548, .T. ) ;
#4208=AXIS2_PLACEMENT_3D ( 'NONE', #3167, #5077, #348 ) ;
#4209=CARTESIAN_POINT ( 'NONE',  ( 12.31015466235495204, 79.04720167209528370, -35.00000000000000711 ) ) ;
#4210=EDGE_CURVE ( 'NONE', #429, #3444, #361, .T. ) ;
#4211=VERTEX_POINT ( 'NONE', #5977 ) ;
#4212=CARTESIAN_POINT ( 'NONE',  ( 9.192833548570215285, 59.02994620157096506, -35.00000000000000000 ) ) ;
#4215=DIRECTION ( 'NONE',  ( -0.4999999999999920619, -0.8660254037844432595, 0.000000000000000000 ) ) ;
#4216=AXIS2_PLACEMENT_3D ( 'NONE', #4566, #2014, #1986 ) ;
#4217=DIRECTION ( 'NONE',  ( -0.000000000000000000, -0.000000000000000000, -1.000000000000000000 ) ) ;
#4218=VECTOR ( 'NONE', #2361, 1000.000000000000000 ) ;
#4222=CIRCLE ( 'NONE', #969, 72.00000000000004263 ) ;
#4223=LINE ( 'NONE', #4190, #5063 ) ;
#4225=ORIENTED_EDGE ( 'NONE', *, *, #2665, .F. ) ;
#4226=ORIENTED_EDGE ( 'NONE', *, *, #2520, .T. ) ;
#4227=CARTESIAN_POINT ( 'NONE',  ( 52.58482424179643289, 72.37680137756268550, -40.00000000000000000 ) ) ;
#4230=DIRECTION ( 'NONE',  ( 0.000000000000000000, -0.000000000000000000, -1.000000000000000000 ) ) ;
#4232=CYLINDRICAL_SURFACE ( 'NONE', #4972, 5.000000000000004441 ) ;
#4233=ORIENTED_EDGE ( 'NONE', *, *, #3275, .T. ) ;
#4237=EDGE_LOOP ( 'NONE', ( #3988, #5618, #1658, #1379, #152 ) ) ;
#4239=EDGE_CURVE ( 'NONE', #2445, #730, #163, .T. ) ;
#4240=ORIENTED_EDGE ( 'NONE', *, *, #4677, .F. ) ;
#4244=AXIS2_PLACEMENT_3D ( 'NONE', #5557, #5148, #2713 ) ;
#4245=DIRECTION ( 'NONE',  ( -0.5000000000000038858, 0.8660254037844362651, 0.000000000000000000 ) ) ;
#4247=AXIS2_PLACEMENT_3D ( 'NONE', #448, #890, #2237 ) ;
#4249=EDGE_CURVE ( 'NONE', #906, #1548, #571, .T. ) ;
#4250=AXIS2_PLACEMENT_3D ( 'NONE', #883, #831, #800 ) ;
#4251=VECTOR ( 'NONE', #3425, 999.9999999999998863 ) ;
#4252=LINE ( 'NONE', #5321, #2764 ) ;
#4255=CONICAL_SURFACE ( 'NONE', #398, 99.00000000000005684, 0.7853981633974552734 ) ;
#4259=ORIENTED_EDGE ( 'NONE', *, *, #1188, .T. ) ;
#4260=EDGE_CURVE ( 'NONE', #2151, #5943, #3438, .T. ) ;
#4265=ORIENTED_EDGE ( 'NONE', *, *, #1777, .T. ) ;
#4267=DIRECTION ( 'NONE',  ( -0.9326495259660420034, -0.3607836771741717574, 0.000000000000000000 ) ) ;
#4270=EDGE_CURVE ( 'NONE', #5854, #5996, #4545, .T. ) ;
#4271=CYLINDRICAL_SURFACE ( 'NONE', #611, 12.50000000000139266 ) ;
#4276=CARTESIAN_POINT ( 'NONE',  ( -80.00000000000000000, 0.000000000000000000, -35.00000000000000000 ) ) ;
#4277=ORIENTED_EDGE ( 'NONE', *, *, #5766, .F. ) ;
#4278=LINE ( 'NONE', #29, #456 ) ;
#4279=CARTESIAN_POINT ( 'NONE',  ( 80.00000000000000000, 0.000000000000000000, 38.99999999999995737 ) ) ;
#4282=DIRECTION ( 'NONE',  ( 1.000000000000000000, 0.000000000000000000, 0.000000000000000000 ) ) ;
#4283=VERTEX_POINT ( 'NONE', #4353 ) ;
#4284=CARTESIAN_POINT ( 'NONE',  ( -9.074396217167167933, -58.26942451214404173, 35.00000000000000000 ) ) ;
#4287=CARTESIAN_POINT ( 'NONE',  ( -7.182140071210238271E-14, 8.916303653273167033E-14, 35.00000000000000000 ) ) ;
#4288=ORIENTED_EDGE ( 'NONE', *, *, #5954, .T. ) ;
#4291=ORIENTED_EDGE ( 'NONE', *, *, #3247, .T. ) ;
#4293=CARTESIAN_POINT ( 'NONE',  ( -52.58482424179695158, -72.37680137756228760, -40.00000000000000000 ) ) ;
#4294=ADVANCED_FACE ( 'NONE', ( #286 ), #2988, .F. ) ;
#4296=CYLINDRICAL_SURFACE ( 'NONE', #790, 4.999999999999997335 ) ;
#4297=CARTESIAN_POINT ( 'NONE',  ( -85.08403291566554572, 27.64547812922971914, -79.99999999999998579 ) ) ;
#4299=VERTEX_POINT ( 'NONE', #1041 ) ;
#4300=EDGE_CURVE ( 'NONE', #3800, #6084, #4923, .T. ) ;
#4309=TOROIDAL_SURFACE ( 'NONE', #5120, 72.00000000000004263, 10.00000000000000000 ) ;
#4312=VERTEX_POINT ( 'NONE', #106 ) ;
#4318=CARTESIAN_POINT ( 'NONE',  ( 5.000000000000003553, 89.46264649666795776, 40.00000000000000000 ) ) ;
#4320=CIRCLE ( 'NONE', #270, 5.000000000000004441 ) ;
#4322=DIRECTION ( 'NONE',  ( 0.4999999999999980016, 0.8660254037844398178, 0.000000000000000000 ) ) ;
#4323=ORIENTED_EDGE ( 'NONE', *, *, #961, .F. ) ;
#4325=CARTESIAN_POINT ( 'NONE',  ( 45.92560378283280187, 36.99336990414421678, 35.00000000000000000 ) ) ;
#4328=AXIS2_PLACEMENT_3D ( 'NONE', #220, #1684, #5969 ) ;
#4329=DIRECTION ( 'NONE',  ( -1.000000000000000000, 0.000000000000000000, 0.000000000000000000 ) ) ;
#4332=ADVANCED_FACE ( 'NONE', ( #2350 ), #4113, .F. ) ;
#4334=ORIENTED_EDGE ( 'NONE', *, *, #1885, .F. ) ;
#4337=CARTESIAN_POINT ( 'NONE',  ( -68.69027832784050247, 26.57196568621489163, 35.13717928826310555 ) ) ;
#4338=ORIENTED_EDGE ( 'NONE', *, *, #128, .T. ) ;
#4339=EDGE_CURVE ( 'NONE', #1288, #5804, #2732, .T. ) ;
#4340=DIRECTION ( 'NONE',  ( 0.4999999999999979461, 0.8660254037844397068, 0.000000000000000000 ) ) ;
#4341=EDGE_CURVE ( 'NONE', #1931, #4450, #1069, .T. ) ;
#4344=ADVANCED_FACE ( 'NONE', ( #1841 ), #3652, .T. ) ;
#4345=DIRECTION ( 'NONE',  ( -0.000000000000000000, -0.000000000000000000, -1.000000000000000000 ) ) ;
#4348=ORIENTED_EDGE ( 'NONE', *, *, #5828, .T. ) ;
#4349=CARTESIAN_POINT ( 'NONE',  ( -67.48246767247867695, 25.10212255632726297, 35.00000000000000000 ) ) ;
#4350=CARTESIAN_POINT ( 'NONE',  ( -68.69027832783800136, -26.57196568621473531, 35.00000000000000000 ) ) ;
#4351=VECTOR ( 'NONE', #2523, 1000.000000000000000 ) ;
#4352=VECTOR ( 'NONE', #4007, 999.9999999999998863 ) ;
#4353=CARTESIAN_POINT ( 'NONE',  ( -55.71784976887420271, -21.55374571496209057, 35.00000000000000000 ) ) ;
#4357=VERTEX_POINT ( 'NONE', #5659 ) ;
#4359=ORIENTED_EDGE ( 'NONE', *, *, #3266, .T. ) ;
#4360=DIRECTION ( 'NONE',  ( 0.000000000000000000, 0.000000000000000000, 1.000000000000000000 ) ) ;
#4362=DIRECTION ( 'NONE',  ( 1.000000000000000000, 0.000000000000000000, 0.000000000000000000 ) ) ;
#4364=AXIS2_PLACEMENT_3D ( 'NONE', #4905, #2111, #2084 ) ;
#4365=LINE ( 'NONE', #1590, #2770 ) ;
#4373=ORIENTED_EDGE ( 'NONE', *, *, #4916, .T. ) ;
#4380=DIRECTION ( 'NONE',  ( 0.6273063437270329779, -0.7787725926866080339, 0.000000000000000000 ) ) ;
#4382=DIRECTION ( 'NONE',  ( -0.000000000000000000, -0.000000000000000000, -1.000000000000000000 ) ) ;
#4383=EDGE_CURVE ( 'NONE', #37, #4784, #5333, .T. ) ;
#4384=PLANE ( 'NONE',  #5651 ) ;
#4385=CARTESIAN_POINT ( 'NONE',  ( 11.33314185116896589, 72.77350886803867525, 35.13717928826270054 ) ) ;
#4387=LINE ( 'NONE', #5919, #2174 ) ;
#4390=DIRECTION ( 'NONE',  ( 0.000000000000000000, 0.000000000000000000, 1.000000000000000000 ) ) ;
#4391=ORIENTED_EDGE ( 'NONE', *, *, #3414, .F. ) ;
#4392=DIRECTION ( 'NONE',  ( -4.496403249731883200E-15, 1.000000000000000000, 0.000000000000000000 ) ) ;
#4393=DIRECTION ( 'NONE',  ( 0.000000000000000000, 0.000000000000000000, 1.000000000000000000 ) ) ;
#4395=DIRECTION ( 'NONE',  ( -0.000000000000000000, -0.000000000000000000, 1.000000000000000000 ) ) ;
#4396=DIRECTION ( 'NONE',  ( 0.000000000000000000, 0.000000000000000000, 1.000000000000000000 ) ) ;
#4400=DIRECTION ( 'NONE',  ( 1.000000000000000000, 0.000000000000000000, 0.000000000000000000 ) ) ;
#4402=CARTESIAN_POINT ( 'NONE',  ( -58.45671475544946816, -33.75000000000027711, 35.00000000000000000 ) ) ;
#4404=APPLICATION_CONTEXT ( 'automotive_design' ) ;
#4405=VERTEX_POINT ( 'NONE', #1382 ) ;
#4407=EDGE_CURVE ( 'NONE', #4299, #993, #4320, .T. ) ;
#4408=EDGE_CURVE ( 'NONE', #413, #2346, #3818, .T. ) ;
#4411=ORIENTED_EDGE ( 'NONE', *, *, #4727, .T. ) ;
#4413=CARTESIAN_POINT ( 'NONE',  ( -52.58482424179695158, -72.37680137756228760, 40.00000000000000000 ) ) ;
#4415=ADVANCED_FACE ( 'NONE', ( #5619 ), #3164, .F. ) ;
#4416=CIRCLE ( 'NONE', #2342, 80.00000000000000000 ) ;
#4418=ORIENTED_EDGE ( 'NONE', *, *, #2780, .F. ) ;
#4420=CIRCLE ( 'NONE', #954, 12.50000000000000178 ) ;
#4421=ORIENTED_EDGE ( 'NONE', *, *, #787, .T. ) ;
#4422=DIRECTION ( 'NONE',  ( 0.000000000000000000, 0.000000000000000000, 1.000000000000000000 ) ) ;
#4423=CARTESIAN_POINT ( 'NONE',  ( -90.08403291566554572, 27.64547812922971914, -79.99999999999998579 ) ) ;
#4425=CARTESIAN_POINT ( 'NONE',  ( -5.000000000000629718, -89.46264649666795776, 40.00000000000000000 ) ) ;
#4426=DIRECTION ( 'NONE',  ( -0.000000000000000000, -0.000000000000000000, 1.000000000000000000 ) ) ;
#4427=AXIS2_PLACEMENT_3D ( 'NONE', #4795, #3323, #4766 ) ;
#4429=ORIENTED_EDGE ( 'NONE', *, *, #2015, .F. ) ;
#4432=DIRECTION ( 'NONE',  ( -0.000000000000000000, -0.000000000000000000, -1.000000000000000000 ) ) ;
#4433=AXIS2_PLACEMENT_3D ( 'NONE', #3312, #2384, #6033 ) ;
#4434=AXIS2_PLACEMENT_3D ( 'NONE', #4177, #3287, #5074 ) ;
#4435=ORIENTED_EDGE ( 'NONE', *, *, #5626, .T. ) ;
#4436=FACE_OUTER_BOUND ( 'NONE', #199, .T. ) ;
#4440=CIRCLE ( 'NONE', #5140, 100.0000000000000000 ) ;
#4442=ORIENTED_EDGE ( 'NONE', *, *, #946, .T. ) ;
#4443=CARTESIAN_POINT ( 'NONE',  ( -55.48030965893044453, 45.89047003626346566, 35.00000000000000000 ) ) ;
#4444=VECTOR ( 'NONE', #339, 1000.000000000000114 ) ;
#4445=EDGE_CURVE ( 'NONE', #4784, #6084, #1754, .T. ) ;
#4446=EDGE_CURVE ( 'NONE', #2223, #3051, #4121, .T. ) ;
#4447=CARTESIAN_POINT ( 'NONE',  ( -68.69027832783800136, -26.57196568621473531, 35.13717928826270054 ) ) ;
#4450=VERTEX_POINT ( 'NONE', #845 ) ;
#4452=ORIENTED_EDGE ( 'NONE', *, *, #3282, .F. ) ;
#4453=CARTESIAN_POINT ( 'NONE',  ( -1.630640067418198669E-13, 67.50000000000002842, 35.00000000000000000 ) ) ;
#4454=DIRECTION ( 'NONE',  ( -0.000000000000000000, 0.000000000000000000, 1.000000000000000000 ) ) ;
#4457=EDGE_CURVE ( 'NONE', #4357, #1548, #2721, .T. ) ;
#4460=AXIS2_PLACEMENT_3D ( 'NONE', #4126, #1760, #3659 ) ;
#4461=EDGE_LOOP ( 'NONE', ( #1219, #4833 ) ) ;
#4462=FACE_OUTER_BOUND ( 'NONE', #2513, .T. ) ;
#4463=CIRCLE ( 'NONE', #3657, 12.50000000000138911 ) ;
#4465=CARTESIAN_POINT ( 'NONE',  ( 7.182140071210238271E-14, -8.916303653273167033E-14, 35.00000000000000000 ) ) ;
#4466=EDGE_CURVE ( 'NONE', #2239, #5444, #1445, .T. ) ;
#4468=DIRECTION ( 'NONE',  ( -0.9326495259660445569, -0.3607836771741652071, 0.000000000000000000 ) ) ;
#4469=B_SPLINE_CURVE_WITH_KNOTS ( 'NONE', 3,
 ( #2143, #2731, #5959, #4577 ),
 .UNSPECIFIED., .F., .F.,
 ( 4, 4 ),
 ( 0.000000000000000000, 0.001907370850886561109 ),
 .UNSPECIFIED. ) ;
#4471=VERTEX_POINT ( 'NONE', #1939 ) ;
#4472=FACE_BOUND ( 'NONE', #4705, .T. ) ;
#4474=DIRECTION ( 'NONE',  ( -0.1538769332794418798, 0.9880900209011901358, 0.000000000000000000 ) ) ;
#4475=ORIENTED_EDGE ( 'NONE', *, *, #138, .T. ) ;
#4477=CARTESIAN_POINT ( 'NONE',  ( 11.07913919611939058, 71.14248150488579370, 45.00000000000000711 ) ) ;
#4482=CARTESIAN_POINT ( 'NONE',  ( 0.000000000000000000, 0.000000000000000000, 35.00000000000000000 ) ) ;
#4483=FACE_OUTER_BOUND ( 'NONE', #1837, .T. ) ;
#4485=DIRECTION ( 'NONE',  ( -0.000000000000000000, -0.000000000000000000, -1.000000000000000000 ) ) ;
#4486=DIRECTION ( 'NONE',  ( -0.000000000000000000, -0.000000000000000000, -1.000000000000000000 ) ) ;
#4487=ORIENTED_EDGE ( 'NONE', *, *, #1487, .T. ) ;
#4488=ADVANCED_FACE ( 'NONE', ( #3404 ), #3772, .F. ) ;
#4492=FACE_OUTER_BOUND ( 'NONE', #5974, .T. ) ;
#4493=EDGE_LOOP ( 'NONE', ( #4883, #5523, #3830, #5288, #5050, #2598, #2628, #2043, #3134, #3363 ) ) ;
#4494=FACE_OUTER_BOUND ( 'NONE', #1045, .T. ) ;
#4495=EDGE_CURVE ( 'NONE', #4527, #5114, #5729, .T. ) ;
#4497=EDGE_LOOP ( 'NONE', ( #5069, #2700, #4721, #4348, #622 ) ) ;
#4499=DIRECTION ( 'NONE',  ( 1.000000000000000000, 0.000000000000000000, 0.000000000000000000 ) ) ;
#4501=LINE ( 'NONE', #5949, #570 ) ;
#4502=EDGE_LOOP ( 'NONE', ( #6139, #938 ) ) ;
#4503=ORIENTED_EDGE ( 'NONE', *, *, #4260, .F. ) ;
#4505=ORIENTED_EDGE ( 'NONE', *, *, #4206, .T. ) ;
#4507=ORIENTED_EDGE ( 'NONE', *, *, #3494, .F. ) ;
#4509=ADVANCED_FACE ( 'NONE', ( #637 ), #4815, .F. ) ;
#4510=DIRECTION ( 'NONE',  ( 0.7787725926866080339, 0.6273063437270329779, 0.000000000000000000 ) ) ;
#4512=DIRECTION ( 'NONE',  ( -0.9880900209011910240, 0.1538769332794358846, 0.000000000000000000 ) ) ;
#4513=DIRECTION ( 'NONE',  ( 0.000000000000000000, 0.000000000000000000, 1.000000000000000000 ) ) ;
#4514=VECTOR ( 'NONE', #3554, 1000.000000000000000 ) ;
#4515=EDGE_LOOP ( 'NONE', ( #352, #784, #3894, #1977 ) ) ;
#4518=DIRECTION ( 'NONE',  ( -0.6273063437270329779, 0.7787725926866080339, 0.000000000000000000 ) ) ;
#4519=CIRCLE ( 'NONE', #58, 12.50000000000138911 ) ;
#4520=EDGE_CURVE ( 'NONE', #1681, #5256, #2942, .T. ) ;
#4523=VERTEX_POINT ( 'NONE', #5688 ) ;
#4524=CARTESIAN_POINT ( 'NONE',  ( -2.941541598353333735E-14, 7.604078429494112756E-14, 35.00000000000000000 ) ) ;
#4526=CIRCLE ( 'NONE', #1634, 5.000000000000005329 ) ;
#4527=VERTEX_POINT ( 'NONE', #963 ) ;
#4528=VECTOR ( 'NONE', #5716, 1000.000000000000000 ) ;
#4530=PLANE ( 'NONE',  #6024 ) ;
#4531=EDGE_CURVE ( 'NONE', #1185, #4450, #3441, .T. ) ;
#4532=CARTESIAN_POINT ( 'NONE',  ( -2.941541598353333735E-14, 7.604078429494112756E-14, -35.00000000000000000 ) ) ;
#4534=DIRECTION ( 'NONE',  ( -0.000000000000000000, 0.000000000000000000, 1.000000000000000000 ) ) ;
#4535=ORIENTED_EDGE ( 'NONE', *, *, #4210, .F. ) ;
#4542=ORIENTED_EDGE ( 'NONE', *, *, #3885, .F. ) ;
#4543=DIRECTION ( 'NONE',  ( 0.7787725926866080339, 0.6273063437270329779, 0.000000000000000000 ) ) ;
#4544=LINE ( 'NONE', #300, #2756 ) ;
#4545=B_SPLINE_CURVE_WITH_KNOTS ( 'NONE', 3,
 ( #3416, #135, #1690, #4385 ),
 .UNSPECIFIED., .F., .F.,
 ( 4, 4 ),
 ( 0.000000000000000000, 0.001907370850883695563 ),
 .UNSPECIFIED. ) ;
#4546=CIRCLE ( 'NONE', #5451, 5.000000000000005329 ) ;
#4547=CARTESIAN_POINT ( 'NONE',  ( -62.30180741492871022, -50.18450749816254586, -35.00000000000000000 ) ) ;
#4552=DIRECTION ( 'NONE',  ( -0.000000000000000000, -0.000000000000000000, 1.000000000000000000 ) ) ;
#4554=CARTESIAN_POINT ( 'NONE',  ( -5.000000000000629718, -89.46264649666795776, -40.00000000000000000 ) ) ;
#4555=CIRCLE ( 'NONE', #1859, 80.00000000000000000 ) ;
#4558=AXIS2_PLACEMENT_3D ( 'NONE', #4227, #5675, #1960 ) ;
#4562=ORIENTED_EDGE ( 'NONE', *, *, #2284, .F. ) ;
#4564=EDGE_CURVE ( 'NONE', #3836, #4690, #3232, .T. ) ;
#4566=CARTESIAN_POINT ( 'NONE',  ( 0.000000000000000000, 0.000000000000000000, -35.00000000000000000 ) ) ;
#4567=AXIS2_PLACEMENT_3D ( 'NONE', #674, #3505, #230 ) ;
#4568=DIRECTION ( 'NONE',  ( 0.9326495259660445569, 0.3607836771741652626, 0.000000000000000000 ) ) ;
#4570=FACE_OUTER_BOUND ( 'NONE', #1938, .T. ) ;
#4571=ORIENTED_EDGE ( 'NONE', *, *, #1928, .T. ) ;
#4573=EDGE_CURVE ( 'NONE', #4952, #6052, #3422, .T. ) ;
#4576=ORIENTED_EDGE ( 'NONE', *, *, #2852, .T. ) ;
#4577=CARTESIAN_POINT ( 'NONE',  ( 12.00215801354989154, -70.99259259259225985, 35.00000000000000000 ) ) ;
#4578=DIRECTION ( 'NONE',  ( 1.154631945610162802E-14, -1.000000000000000000, 0.000000000000000000 ) ) ;
#4580=DIRECTION ( 'NONE',  ( -0.1538769332794358846, -0.9880900209011910240, 0.000000000000000000 ) ) ;
#4582=DIRECTION ( 'NONE',  ( 1.000000000000000000, 0.000000000000000000, 0.000000000000000000 ) ) ;
#4583=ORIENTED_EDGE ( 'NONE', *, *, #5221, .T. ) ;
#4590=ORIENTED_EDGE ( 'NONE', *, *, #4793, .F. ) ;
#4592=DIRECTION ( 'NONE',  ( 0.000000000000000000, -0.000000000000000000, 1.000000000000000000 ) ) ;
#4595=PLANE ( 'NONE',  #5326 ) ;
#4596=ORIENTED_EDGE ( 'NONE', *, *, #5954, .F. ) ;
#4597=EDGE_CURVE ( 'NONE', #1798, #2346, #538, .T. ) ;
#4598=EDGE_CURVE ( 'NONE', #4357, #4988, #3128, .T. ) ;
#4601=DIRECTION ( 'NONE',  ( 0.7787725926866080339, 0.6273063437270329779, 0.000000000000000000 ) ) ;
#4602=EDGE_LOOP ( 'NONE', ( #5105, #221, #4590, #5354, #4696, #1437 ) ) ;
#4603=LINE ( 'NONE', #4096, #5467 ) ;
#4607=B_SPLINE_CURVE_WITH_KNOTS ( 'NONE', 3,
 ( #1456, #5170, #5270, #975 ),
 .UNSPECIFIED., .F., .F.,
 ( 4, 4 ),
 ( 0.000000000000000000, 0.001907370850886568915 ),
 .UNSPECIFIED. ) ;
#4608=FACE_OUTER_BOUND ( 'NONE', #3979, .T. ) ;
#4609=CARTESIAN_POINT ( 'NONE',  ( -52.58482424179536707, 72.37680137756343868, 40.00000000000000000 ) ) ;
#4610=EDGE_LOOP ( 'NONE', ( #419, #5251, #3630, #5360 ) ) ;
#4612=LINE ( 'NONE', #2242, #3521 ) ;
#4616=ORIENTED_EDGE ( 'NONE', *, *, #2781, .F. ) ;
#4618=CARTESIAN_POINT ( 'NONE',  ( 80.99999999999998579, 9.919639073093559622E-15, -40.00000000000000000 ) ) ;
#4620=CIRCLE ( 'NONE', #4427, 99.00000000000000000 ) ;
#4621=DIRECTION ( 'NONE',  ( 0.000000000000000000, 0.000000000000000000, 1.000000000000000000 ) ) ;
#4622=CIRCLE ( 'NONE', #1068, 10.00000000000000000 ) ;
#4624=ADVANCED_FACE ( 'NONE', ( #4889 ), #92, .F. ) ;
#4626=DIRECTION ( 'NONE',  ( 0.000000000000000000, 0.000000000000000000, 1.000000000000000000 ) ) ;
#4627=AXIS2_PLACEMENT_3D ( 'NONE', #2938, #660, #1121 ) ;
#4628=CIRCLE ( 'NONE', #68, 4.999999999999997335 ) ;
#4629=AXIS2_PLACEMENT_3D ( 'NONE', #5076, #4152, #877 ) ;
#4632=ORIENTED_EDGE ( 'NONE', *, *, #6122, .T. ) ;
#4633=DIRECTION ( 'NONE',  ( 1.000000000000000000, 0.000000000000000000, 0.000000000000000000 ) ) ;
#4634=ORIENTED_EDGE ( 'NONE', *, *, #1266, .F. ) ;
#4635=CARTESIAN_POINT ( 'NONE',  ( 0.000000000000000000, 0.000000000000000000, 38.99999999999995737 ) ) ;
#4636=EDGE_CURVE ( 'NONE', #5346, #2846, #4278, .T. ) ;
#4637=DIRECTION ( 'NONE',  ( 1.000000000000000000, 0.000000000000000000, 0.000000000000000000 ) ) ;
#4640=CARTESIAN_POINT ( 'NONE',  ( -47.58482424179536707, 72.37680137756343868, 40.00000000000000000 ) ) ;
#4643=EDGE_CURVE ( 'NONE', #3297, #559, #1906, .T. ) ;
#4644=DIRECTION ( 'NONE',  ( -0.000000000000000000, -0.000000000000000000, 1.000000000000000000 ) ) ;
#4645=DIRECTION ( 'NONE',  ( -0.7787725926866080339, -0.6273063437270329779, 0.000000000000000000 ) ) ;
#4649=ORIENTED_EDGE ( 'NONE', *, *, #3873, .F. ) ;
#4652=AXIS2_PLACEMENT_3D ( 'NONE', #3410, #5322, #614 ) ;
#4653=CARTESIAN_POINT ( 'NONE',  ( -12.00215801354769063, -70.99259259259262933, 35.00000000000000000 ) ) ;
#4654=VECTOR ( 'NONE', #1430, 1000.000000000000000 ) ;
#4656=DIRECTION ( 'NONE',  ( 0.7787725926866119197, -0.6273063437270283149, 0.000000000000000000 ) ) ;
#4657=VECTOR ( 'NONE', #5265, 1000.000000000000000 ) ;
#4660=CARTESIAN_POINT ( 'NONE',  ( -6.247143215332724651E-13, -89.46264649666795776, -40.00000000000000000 ) ) ;
#4661=AXIS2_PLACEMENT_3D ( 'NONE', #1925, #5780, #2996 ) ;
#4663=ORIENTED_EDGE ( 'NONE', *, *, #3439, .F. ) ;
#4666=DIRECTION ( 'NONE',  ( 0.000000000000000000, 0.000000000000000000, 1.000000000000000000 ) ) ;
#4667=DIRECTION ( 'NONE',  ( 1.000000000000000000, 0.000000000000000000, 0.000000000000000000 ) ) ;
#4668=LINE ( 'NONE', #5731, #3522 ) ;
#4671=CARTESIAN_POINT ( 'NONE',  ( 2.941541598353386116E-14, -7.604078429494091299E-14, 35.00000000000000000 ) ) ;
#4672=VERTEX_POINT ( 'NONE', #2630 ) ;
#4673=LINE ( 'NONE', #4192, #5358 ) ;
#4674=CARTESIAN_POINT ( 'NONE',  ( -85.08403291566554572, 27.64547812922971914, -79.99999999999998579 ) ) ;
#4675=DIRECTION ( 'NONE',  ( -0.000000000000000000, -0.000000000000000000, -1.000000000000000000 ) ) ;
#4677=EDGE_CURVE ( 'NONE', #1473, #705, #5034, .T. ) ;
#4678=DIRECTION ( 'NONE',  ( 1.000000000000000000, 0.000000000000000000, 0.000000000000000000 ) ) ;
#4681=FACE_OUTER_BOUND ( 'NONE', #2881, .T. ) ;
#4682=ORIENTED_EDGE ( 'NONE', *, *, #1487, .F. ) ;
#4685=ADVANCED_FACE ( 'NONE', ( #4436 ), #3067, .F. ) ;
#4687=CYLINDRICAL_SURFACE ( 'NONE', #3033, 12.50000000000139089 ) ;
#4689=FACE_OUTER_BOUND ( 'NONE', #1391, .T. ) ;
#4690=VERTEX_POINT ( 'NONE', #2605 ) ;
#4691=DIRECTION ( 'NONE',  ( -0.000000000000000000, -0.000000000000000000, -1.000000000000000000 ) ) ;
#4692=ORIENTED_EDGE ( 'NONE', *, *, #4339, .T. ) ;
#4693=FACE_OUTER_BOUND ( 'NONE', #2171, .T. ) ;
#4696=ORIENTED_EDGE ( 'NONE', *, *, #4520, .T. ) ;
#4697=DIRECTION ( 'NONE',  ( 1.000000000000000000, 0.000000000000000000, 0.000000000000000000 ) ) ;
#4698=CARTESIAN_POINT ( 'NONE',  ( -56.07162667343609286, 45.16605674834606532, 45.00000000000000711 ) ) ;
#4700=ORIENTED_EDGE ( 'NONE', *, *, #241, .F. ) ;
#4701=CARTESIAN_POINT ( 'NONE',  ( 6.314393452555577824E-13, -67.50000000000002842, -35.00000000000000000 ) ) ;
#4705=EDGE_LOOP ( 'NONE', ( #3281, #5589 ) ) ;
#4708=DIRECTION ( 'NONE',  ( -0.000000000000000000, 0.000000000000000000, 1.000000000000000000 ) ) ;
#4709=ADVANCED_FACE ( 'NONE', ( #2066 ), #5940, .F. ) ;
#4710=ADVANCED_FACE ( 'NONE', ( #4494 ), #4309, .F. ) ;
#4711=VERTEX_POINT ( 'NONE', #1207 ) ;
#4715=ADVANCED_FACE ( 'NONE', ( #4977 ), #247, .F. ) ;
#4717=VECTOR ( 'NONE', #4104, 1000.000000000000000 ) ;
#4719=AXIS2_PLACEMENT_3D ( 'NONE', #1855, #5697, #2862 ) ;
#4721=ORIENTED_EDGE ( 'NONE', *, *, #3355, .T. ) ;
#4722=CARTESIAN_POINT ( 'NONE',  ( 52.58482424179591419, -72.37680137756305498, 40.00000000000000000 ) ) ;
#4725=CARTESIAN_POINT ( 'NONE',  ( 0.000000000000000000, 0.000000000000000000, 35.00000000000000000 ) ) ;
#4727=EDGE_CURVE ( 'NONE', #5424, #3675, #5442, .T. ) ;
#4728=DIRECTION ( 'NONE',  ( -0.000000000000000000, -0.000000000000000000, -1.000000000000000000 ) ) ;
#4729=CARTESIAN_POINT ( 'NONE',  ( 80.08403291566574467, -27.64547812922912939, 40.00000000000000000 ) ) ;
#4730=ORIENTED_EDGE ( 'NONE', *, *, #1149, .T. ) ;
#4732=AXIS2_PLACEMENT_3D ( 'NONE', #3469, #1506, #4400 ) ;
#4737=CARTESIAN_POINT ( 'NONE',  ( -11.33314185116958051, 72.77350886804100583, -35.00000000000000000 ) ) ;
#4738=PRODUCT ( 'Roll rack Rotating wheel', 'Roll rack Rotating wheel', '', ( #4009 ) ) ;
#4739=LINE ( 'NONE', #492, #2357 ) ;
#4742=LINE ( 'NONE', #2874, #5873 ) ;
#4745=EDGE_LOOP ( 'NONE', ( #3883, #2584, #5658, #3371 ) ) ;
#4746=AXIS2_PLACEMENT_3D ( 'NONE', #3120, #5029, #2538 ) ;
#4749=CARTESIAN_POINT ( 'NONE',  ( 56.72666074499640843, -46.14586675604078891, 35.04915833130704073 ) ) ;
#4750=ORIENTED_EDGE ( 'NONE', *, *, #2200, .F. ) ;
#4751=DIRECTION ( 'NONE',  ( 1.000000000000000000, 0.000000000000000000, 0.000000000000000000 ) ) ;
#4752=VECTOR ( 'NONE', #386, 1000.000000000000114 ) ;
#4755=AXIS2_PLACEMENT_3D ( 'NONE', #5051, #4038, #2205 ) ;
#4756=FACE_OUTER_BOUND ( 'NONE', #4237, .T. ) ;
#4758=CIRCLE ( 'NONE', #4964, 12.50000000000138911 ) ;
#4762=CIRCLE ( 'NONE', #5068, 80.00000000000000000 ) ;
#4764=CARTESIAN_POINT ( 'NONE',  ( 52.58482424179591419, -72.37680137756305498, -79.99999999999998579 ) ) ;
#4766=DIRECTION ( 'NONE',  ( 1.000000000000000000, 0.000000000000000000, 0.000000000000000000 ) ) ;
#4769=AXIS2_PLACEMENT_3D ( 'NONE', #2016, #1551, #5830 ) ;
#4770=ADVANCED_FACE ( 'NONE', ( #3097 ), #4818, .F. ) ;
#4773=VERTEX_POINT ( 'NONE', #3031 ) ;
#4774=PLANE ( 'NONE',  #3558 ) ;
#4780=ORIENTED_EDGE ( 'NONE', *, *, #4992, .F. ) ;
#4783=DIRECTION ( 'NONE',  ( 0.000000000000000000, 0.000000000000000000, 1.000000000000000000 ) ) ;
#4784=VERTEX_POINT ( 'NONE', #748 ) ;
#4785=CARTESIAN_POINT ( 'NONE',  ( 55.71784976887403928, 21.55374571496248137, 35.00000000000000000 ) ) ;
#4788=DIRECTION ( 'NONE',  ( -0.000000000000000000, -0.000000000000000000, 1.000000000000000000 ) ) ;
#4790=VERTEX_POINT ( 'NONE', #279 ) ;
#4791=DIRECTION ( 'NONE',  ( 0.000000000000000000, 0.000000000000000000, 1.000000000000000000 ) ) ;
#4793=EDGE_CURVE ( 'NONE', #1202, #5854, #5320, .T. ) ;
#4795=CARTESIAN_POINT ( 'NONE',  ( 0.000000000000000000, 0.000000000000000000, -40.00000000000000000 ) ) ;
#4799=EDGE_LOOP ( 'NONE', ( #24, #4847 ) ) ;
#4800=ORIENTED_EDGE ( 'NONE', *, *, #5347, .F. ) ;
#4801=DIRECTION ( 'NONE',  ( 0.000000000000000000, 0.000000000000000000, 1.000000000000000000 ) ) ;
#4803=LINE ( 'NONE', #3333, #1563 ) ;
#4805=EDGE_CURVE ( 'NONE', #4299, #3865, #5504, .T. ) ;
#4807=CARTESIAN_POINT ( 'NONE',  ( -7.182140071210238271E-14, 8.916303653273167033E-14, 35.00000000000000000 ) ) ;
#4814=ORIENTED_EDGE ( 'NONE', *, *, #4920, .T. ) ;
#4815=PLANE ( 'NONE',  #373 ) ;
#4818=CONICAL_SURFACE ( 'NONE', #1161, 80.99999999999998579, 0.7853981633974482790 ) ;
#4819=DIRECTION ( 'NONE',  ( 1.000000000000000000, 0.000000000000000000, 0.000000000000000000 ) ) ;
#4820=CARTESIAN_POINT ( 'NONE',  ( 56.72666074499684896, 46.14586675604289212, 35.04915833130718994 ) ) ;
#4821=VERTEX_POINT ( 'NONE', #3126 ) ;
#4822=CARTESIAN_POINT ( 'NONE',  ( 0.000000000000000000, 0.000000000000000000, 38.99999999999995737 ) ) ;
#4823=LINE ( 'NONE', #1853, #1757 ) ;
#4825=AXIS2_PLACEMENT_3D ( 'NONE', #238, #3055, #4996 ) ;
#4826=DIRECTION ( 'NONE',  ( -0.000000000000000000, -0.000000000000000000, -1.000000000000000000 ) ) ;
#4827=CARTESIAN_POINT ( 'NONE',  ( -9.192833548570215285, -59.02994620157096506, 35.00000000000000000 ) ) ;
#4830=AXIS2_PLACEMENT_3D ( 'NONE', #30, #3804, #2790 ) ;
#4831=AXIS2_PLACEMENT_3D ( 'NONE', #2486, #3376, #2446 ) ;
#4833=ORIENTED_EDGE ( 'NONE', *, *, #4091, .T. ) ;
#4834=CARTESIAN_POINT ( 'NONE',  ( 90.08403291566594362, 27.64547812922851833, -40.00000000000000000 ) ) ;
#4835=VERTEX_POINT ( 'NONE', #2572 ) ;
#4836=DIRECTION ( 'NONE',  ( -0.000000000000000000, 0.000000000000000000, 1.000000000000000000 ) ) ;
#4837=FACE_OUTER_BOUND ( 'NONE', #2006, .T. ) ;
#4839=AXIS2_PLACEMENT_3D ( 'NONE', #1652, #4432, #2063 ) ;
#4841=VECTOR ( 'NONE', #693, 1000.000000000000000 ) ;
#4843=ORIENTED_EDGE ( 'NONE', *, *, #154, .T. ) ;
#4844=EDGE_CURVE ( 'NONE', #2998, #5851, #3025, .T. ) ;
#4847=ORIENTED_EDGE ( 'NONE', *, *, #5897, .T. ) ;
#4850=CARTESIAN_POINT ( 'NONE',  ( 0.000000000000000000, 0.000000000000000000, -40.00000000000000000 ) ) ;
#4851=AXIS2_PLACEMENT_3D ( 'NONE', #5422, #4036, #762 ) ;
#4852=ORIENTED_EDGE ( 'NONE', *, *, #4677, .T. ) ;
#4853=DIRECTION ( 'NONE',  ( 0.000000000000000000, -0.000000000000000000, 1.000000000000000000 ) ) ;
#4856=ADVANCED_FACE ( 'NONE', ( #4462 ), #5935, .F. ) ;
#4858=VERTEX_POINT ( 'NONE', #1650 ) ;
#4860=VECTOR ( 'NONE', #5465, 1000.000000000000000 ) ;
#4864=EDGE_LOOP ( 'NONE', ( #2768, #4937, #4507, #5889, #5217, #5387, #2457, #4277 ) ) ;
#4865=CARTESIAN_POINT ( 'NONE',  ( 85.08403291566592941, 27.64547812922851833, 40.00000000000000000 ) ) ;
#4870=ORIENTED_EDGE ( 'NONE', *, *, #3752, .T. ) ;
#4871=AXIS2_PLACEMENT_3D ( 'NONE', #5901, #4396, #2967 ) ;
#4873=ORIENTED_EDGE ( 'NONE', *, *, #3003, .T. ) ;
#4874=CARTESIAN_POINT ( 'NONE',  ( -68.69027832783800136, -26.57196568621473531, -35.00000000000000000 ) ) ;
#4875=ORIENTED_EDGE ( 'NONE', *, *, #5522, .T. ) ;
#4876=CARTESIAN_POINT ( 'NONE',  ( -85.08403291566612836, -27.64547812922793923, -40.00000000000000000 ) ) ;
#4879=VECTOR ( 'NONE', #143, 1000.000000000000114 ) ;
#4881=DIRECTION ( 'NONE',  ( 1.000000000000000000, 0.000000000000000000, 0.000000000000000000 ) ) ;
#4883=ORIENTED_EDGE ( 'NONE', *, *, #5617, .F. ) ;
#4886=DIRECTION ( 'NONE',  ( 0.000000000000000000, 0.000000000000000000, 1.000000000000000000 ) ) ;
#4889=FACE_OUTER_BOUND ( 'NONE', #228, .T. ) ;
#4895=CARTESIAN_POINT ( 'NONE',  ( 47.58482424179642578, 72.37680137756268550, -79.99999999999998579 ) ) ;
#4896=EDGE_LOOP ( 'NONE', ( #5476, #4391, #4147, #4411 ) ) ;
#4897=LINE ( 'NONE', #3975, #3936 ) ;
#4900=VERTEX_POINT ( 'NONE', #2188 ) ;
#4902=ORIENTED_EDGE ( 'NONE', *, *, #4916, .F. ) ;
#4904=CARTESIAN_POINT ( 'NONE',  ( 2.941541598353386116E-14, -7.604078429494091299E-14, 35.00000000000000000 ) ) ;
#4905=CARTESIAN_POINT ( 'NONE',  ( 58.45671475544992290, -33.74999999999945999, 35.00000000000000000 ) ) ;
#4906=CARTESIAN_POINT ( 'NONE',  ( 85.08403291566592941, 27.64547812922851833, -79.99999999999998579 ) ) ;
#4907=EDGE_LOOP ( 'NONE', ( #2360, #5033 ) ) ;
#4908=EDGE_CURVE ( 'NONE', #5243, #1713, #3000, .T. ) ;
#4912=PLANE ( 'NONE',  #4627 ) ;
#4913=ORIENTED_EDGE ( 'NONE', *, *, #1188, .F. ) ;
#4915=ORIENTED_EDGE ( 'NONE', *, *, #4098, .F. ) ;
#4916=EDGE_CURVE ( 'NONE', #5574, #15, #2326, .T. ) ;
#4917=EDGE_CURVE ( 'NONE', #5256, #1713, #658, .T. ) ;
#4920=EDGE_CURVE ( 'NONE', #6052, #4952, #4628, .T. ) ;
#4921=ORIENTED_EDGE ( 'NONE', *, *, #5007, .F. ) ;
#4922=DIRECTION ( 'NONE',  ( 0.000000000000000000, 0.000000000000000000, 1.000000000000000000 ) ) ;
#4923=LINE ( 'NONE', #2917, #4021 ) ;
#4924=FACE_BOUND ( 'NONE', #5673, .T. ) ;
#4926=ADVANCED_FACE ( 'NONE', ( #3697 ), #364, .F. ) ;
#4927=EDGE_LOOP ( 'NONE', ( #4225, #5950 ) ) ;
#4931=DIRECTION ( 'NONE',  ( 0.000000000000000000, 0.000000000000000000, 1.000000000000000000 ) ) ;
#4932=DIRECTION ( 'NONE',  ( -0.000000000000000000, -0.000000000000000000, -1.000000000000000000 ) ) ;
#4934=DIRECTION ( 'NONE',  ( -0.000000000000000000, -0.000000000000000000, 1.000000000000000000 ) ) ;
#4935=DIRECTION ( 'NONE',  ( -0.1538769332794418798, 0.9880900209011901358, 0.000000000000000000 ) ) ;
#4936=AXIS2_PLACEMENT_3D ( 'NONE', #5468, #5429, #2024 ) ;
#4937=ORIENTED_EDGE ( 'NONE', *, *, #5486, .F. ) ;
#4942=AXIS2_PLACEMENT_3D ( 'NONE', #4150, #6064, #1785 ) ;
#4945=PRODUCT_DEFINITION_FORMATION_WITH_SPECIFIED_SOURCE ( 'ANY', '', #4738, .NOT_KNOWN. ) ;
#4947=ORIENTED_EDGE ( 'NONE', *, *, #1625, .T. ) ;
#4948=CIRCLE ( 'NONE', #4851, 80.00000000000000000 ) ;
#4949=DIRECTION ( 'NONE',  ( -0.000000000000000000, 0.000000000000000000, 1.000000000000000000 ) ) ;
#4951=CARTESIAN_POINT ( 'NONE',  ( -67.15076586955559890, 25.97642475653904270, 45.00000000000000711 ) ) ;
#4952=VERTEX_POINT ( 'NONE', #921 ) ;
#4953=DIRECTION ( 'NONE',  ( 1.000000000000000000, 0.000000000000000000, 0.000000000000000000 ) ) ;
#4954=EDGE_CURVE ( 'NONE', #1931, #2370, #3276, .T. ) ;
#4960=VERTEX_POINT ( 'NONE', #3210 ) ;
#4961=CARTESIAN_POINT ( 'NONE',  ( -80.08403291566614257, -27.64547812922793923, -40.00000000000000000 ) ) ;
#4964=AXIS2_PLACEMENT_3D ( 'NONE', #4453, #4991, #3950 ) ;
#4965=CARTESIAN_POINT ( 'NONE',  ( 57.35713647666955950, -46.20154318182373032, 35.13717928826270054 ) ) ;
#4967=CARTESIAN_POINT ( 'NONE',  ( 8.056095891487838412E-14, -1.254589464284425060E-14, -35.00000000000000000 ) ) ;
#4970=ORIENTED_EDGE ( 'NONE', *, *, #4249, .T. ) ;
#4971=CARTESIAN_POINT ( 'NONE',  ( 0.000000000000000000, 0.000000000000000000, 35.00000000000000000 ) ) ;
#4972=AXIS2_PLACEMENT_3D ( 'NONE', #1899, #5707, #3429 ) ;
#4974=CARTESIAN_POINT ( 'NONE',  ( -27.50000000000000355, -47.63139720814412215, -35.00000000000000000 ) ) ;
#4975=SHAPE_REPRESENTATION ( 'Roll rack Rotating wheel', ( #73 ), #5734 ) ;
#4976=VERTEX_POINT ( 'NONE', #3150 ) ;
#4977=FACE_OUTER_BOUND ( 'NONE', #1761, .T. ) ;
#4979=ORIENTED_EDGE ( 'NONE', *, *, #4954, .T. ) ;
#4982=CYLINDRICAL_SURFACE ( 'NONE', #3437, 5.000000000000004441 ) ;
#4984=VERTEX_POINT ( 'NONE', #2274 ) ;
#4985=PLANE ( 'NONE',  #4567 ) ;
#4988=VERTEX_POINT ( 'NONE', #5558 ) ;
#4990=ORIENTED_EDGE ( 'NONE', *, *, #3455, .F. ) ;
#4991=DIRECTION ( 'NONE',  ( 0.000000000000000000, 0.000000000000000000, 1.000000000000000000 ) ) ;
#4992=EDGE_CURVE ( 'NONE', #3466, #37, #4193, .T. ) ;
#4993=EDGE_CURVE ( 'NONE', #4672, #1816, #4420, .T. ) ;
#4994=CARTESIAN_POINT ( 'NONE',  ( 0.000000000000000000, 0.000000000000000000, 35.00000000000000000 ) ) ;
#4996=DIRECTION ( 'NONE',  ( -1.000000000000000000, 0.000000000000000000, 0.000000000000000000 ) ) ;
#4997=FACE_OUTER_BOUND ( 'NONE', #1091, .T. ) ;
#4998=ORIENTED_EDGE ( 'NONE', *, *, #4844, .F. ) ;
#4999=EDGE_CURVE ( 'NONE', #5202, #2841, #4519, .T. ) ;
#5003=ORIENTED_EDGE ( 'NONE', *, *, #5221, .F. ) ;
#5004=CARTESIAN_POINT ( 'NONE',  ( 8.056095891487838412E-14, -1.254589464284425060E-14, 35.00000000000000000 ) ) ;
#5006=ORIENTED_EDGE ( 'NONE', *, *, #2851, .F. ) ;
#5007=EDGE_CURVE ( 'NONE', #2468, #1974, #155, .T. ) ;
#5008=FACE_BOUND ( 'NONE', #5107, .T. ) ;
#5010=DIRECTION ( 'NONE',  ( -1.000000000000000000, 0.000000000000000000, 0.000000000000000000 ) ) ;
#5011=EDGE_LOOP ( 'NONE', ( #4800, #1536, #5276, #1232 ) ) ;
#5012=ORIENTED_EDGE ( 'NONE', *, *, #2734, .F. ) ;
#5013=CARTESIAN_POINT ( 'NONE',  ( 0.000000000000000000, 67.50000000000000000, -35.00000000000000000 ) ) ;
#5015=VERTEX_POINT ( 'NONE', #1310 ) ;
#5016=CARTESIAN_POINT ( 'NONE',  ( -12.31015466235495204, -79.04720167209528370, -35.00000000000000711 ) ) ;
#5018=CARTESIAN_POINT ( 'NONE',  ( -46.52501622030417394, 37.47620048660903080, 35.00000000000000000 ) ) ;
#5019=DIRECTION ( 'NONE',  ( 0.000000000000000000, 0.000000000000000000, -1.000000000000000000 ) ) ;
#5021=CARTESIAN_POINT ( 'NONE',  ( 0.000000000000000000, -67.50000000000000000, -35.00000000000000000 ) ) ;
#5026=EDGE_LOOP ( 'NONE', ( #1982, #2249, #3354, #1478, #4323, #2616 ) ) ;
#5028=DIRECTION ( 'NONE',  ( 1.000000000000000000, 0.000000000000000000, 0.000000000000000000 ) ) ;
#5029=DIRECTION ( 'NONE',  ( -0.9880900209011902469, -0.1538769332794418798, 0.000000000000000000 ) ) ;
#5030=DIRECTION ( 'NONE',  ( -0.4999999999999918954, -0.8660254037844433705, 0.000000000000000000 ) ) ;
#5031=AXIS2_PLACEMENT_3D ( 'NONE', #2900, #2870, #5279 ) ;
#5033=ORIENTED_EDGE ( 'NONE', *, *, #3275, .F. ) ;
#5034=LINE ( 'NONE', #1598, #4841 ) ;
#5037=AXIS2_PLACEMENT_3D ( 'NONE', #2099, #1179, #5447 ) ;
#5038=ORIENTED_EDGE ( 'NONE', *, *, #130, .F. ) ;
#5040=DIRECTION ( 'NONE',  ( -0.000000000000000000, -0.000000000000000000, 1.000000000000000000 ) ) ;
#5041=CIRCLE ( 'NONE', #2642, 12.49999999999999822 ) ;
#5042=DIRECTION ( 'NONE',  ( 1.000000000000000000, 0.000000000000000000, 0.000000000000000000 ) ) ;
#5044=CARTESIAN_POINT ( 'NONE',  ( -80.08403291566554572, 27.64547812922971914, -40.00000000000000000 ) ) ;
#5050=ORIENTED_EDGE ( 'NONE', *, *, #2230, .F. ) ;
#5051=CARTESIAN_POINT ( 'NONE',  ( -85.08403291566612836, -27.64547812922793923, 40.00000000000000000 ) ) ;
#5052=DIRECTION ( 'NONE',  ( 1.000000000000000000, 0.000000000000000000, 0.000000000000000000 ) ) ;
#5054=DIRECTION ( 'NONE',  ( -1.000000000000000000, 0.000000000000000000, 0.000000000000000000 ) ) ;
#5055=AXIS2_PLACEMENT_3D ( 'NONE', #6109, #6055, #1742 ) ;
#5059=FACE_OUTER_BOUND ( 'NONE', #2440, .T. ) ;
#5063=VECTOR ( 'NONE', #858, 1000.000000000000000 ) ;
#5064=ORIENTED_EDGE ( 'NONE', *, *, #1129, .F. ) ;
#5066=VECTOR ( 'NONE', #6036, 1000.000000000000000 ) ;
#5068=AXIS2_PLACEMENT_3D ( 'NONE', #2185, #1703, #3604 ) ;
#5069=ORIENTED_EDGE ( 'NONE', *, *, #4993, .F. ) ;
#5073=EDGE_CURVE ( 'NONE', #2569, #2065, #3642, .T. ) ;
#5074=DIRECTION ( 'NONE',  ( -0.5000000000000039968, 0.8660254037844363761, 0.000000000000000000 ) ) ;
#5075=VECTOR ( 'NONE', #5342, 1000.000000000000000 ) ;
#5076=CARTESIAN_POINT ( 'NONE',  ( 52.58482424179643289, 72.37680137756268550, 40.00000000000000000 ) ) ;
#5077=DIRECTION ( 'NONE',  ( -0.3607836771741531612, -0.9326495259660493309, 0.000000000000000000 ) ) ;
#5079=EDGE_CURVE ( 'NONE', #1368, #3265, #4612, .T. ) ;
#5081=EDGE_LOOP ( 'NONE', ( #4487, #2113 ) ) ;
#5083=ORIENTED_EDGE ( 'NONE', *, *, #1810, .T. ) ;
#5085=CARTESIAN_POINT ( 'NONE',  ( -58.45671475544962448, -33.75000000000001421, 35.00000000000000000 ) ) ;
#5086=CARTESIAN_POINT ( 'NONE',  ( -12.00215801354939948, 70.99259259259233090, 35.00000000000000000 ) ) ;
#5089=ORIENTED_EDGE ( 'NONE', *, *, #5364, .F. ) ;
#5090=DIRECTION ( 'NONE',  ( 0.1538769332794418798, -0.9880900209011901358, 0.000000000000000000 ) ) ;
#5098=LINE ( 'NONE', #1875, #3037 ) ;
#5099=DIRECTION ( 'NONE',  ( 1.000000000000000000, 0.000000000000000000, 0.000000000000000000 ) ) ;
#5105=ORIENTED_EDGE ( 'NONE', *, *, #128, .F. ) ;
#5106=DIRECTION ( 'NONE',  ( -0.7071067811865474617, 0.000000000000000000, -0.7071067811865474617 ) ) ;
#5107=EDGE_LOOP ( 'NONE', ( #4095, #1890 ) ) ;
#5108=DIRECTION ( 'NONE',  ( -0.9326495259660420034, -0.3607836771741717574, 0.000000000000000000 ) ) ;
#5114=VERTEX_POINT ( 'NONE', #1961 ) ;
#5115=DIRECTION ( 'NONE',  ( 0.000000000000000000, 0.000000000000000000, 1.000000000000000000 ) ) ;
#5120=AXIS2_PLACEMENT_3D ( 'NONE', #1125, #2660, #5852 ) ;
#5122=ORIENTED_EDGE ( 'NONE', *, *, #4300, .F. ) ;
#5124=CARTESIAN_POINT ( 'NONE',  ( 0.000000000000000000, 0.000000000000000000, 40.00000000000000000 ) ) ;
#5126=( GEOMETRIC_REPRESENTATION_CONTEXT ( 3 ) GLOBAL_UNCERTAINTY_ASSIGNED_CONTEXT ( ( #3196 ) ) GLOBAL_UNIT_ASSIGNED_CONTEXT ( ( #3129, #4087, #1076 ) ) REPRESENTATION_CONTEXT ( 'NONE', 'WORKASPACE' ) );
#5127=DIRECTION ( 'NONE',  ( 0.000000000000000000, 0.000000000000000000, 1.000000000000000000 ) ) ;
#5129=AXIS2_PLACEMENT_3D ( 'NONE', #1293, #4621, #5099 ) ;
#5133=AXIS2_PLACEMENT_3D ( 'NONE', #3907, #4922, #5824 ) ;
#5136=ORIENTED_EDGE ( 'NONE', *, *, #5876, .F. ) ;
#5137=CARTESIAN_POINT ( 'NONE',  ( 52.58482424179643289, 72.37680137756268550, -40.00000000000000000 ) ) ;
#5138=VERTEX_POINT ( 'NONE', #1403 ) ;
#5140=AXIS2_PLACEMENT_3D ( 'NONE', #589, #2467, #4678 ) ;
#5142=EDGE_CURVE ( 'NONE', #4450, #5737, #3859, .T. ) ;
#5147=ORIENTED_EDGE ( 'NONE', *, *, #324, .F. ) ;
#5148=DIRECTION ( 'NONE',  ( -0.000000000000000000, -0.000000000000000000, 1.000000000000000000 ) ) ;
#5150=EDGE_CURVE ( 'NONE', #4960, #2272, #3502, .T. ) ;
#5154=AXIS2_PLACEMENT_3D ( 'NONE', #3881, #913, #3267 ) ;
#5155=ORIENTED_EDGE ( 'NONE', *, *, #3600, .F. ) ;
#5159=VECTOR ( 'NONE', #4392, 1000.000000000000000 ) ;
#5160=ORIENTED_EDGE ( 'NONE', *, *, #4564, .F. ) ;
#5161=DIRECTION ( 'NONE',  ( 1.000000000000000000, 0.000000000000000000, 0.000000000000000000 ) ) ;
#5162=VECTOR ( 'NONE', #182, 1000.000000000000000 ) ;
#5163=CARTESIAN_POINT ( 'NONE',  ( 0.000000000000000000, 0.000000000000000000, -39.00000000000001421 ) ) ;
#5168=CARTESIAN_POINT ( 'NONE',  ( 52.58482424179591419, -72.37680137756305498, 40.00000000000000000 ) ) ;
#5169=EDGE_LOOP ( 'NONE', ( #524, #2114, #107, #1030 ) ) ;
#5170=CARTESIAN_POINT ( 'NONE',  ( 68.32682326288367847, -26.05379589900651638, 35.04915833130718994 ) ) ;
#5171=DIRECTION ( 'NONE',  ( -0.000000000000000000, -0.000000000000000000, -1.000000000000000000 ) ) ;
#5172=ORIENTED_EDGE ( 'NONE', *, *, #3529, .T. ) ;
#5173=DIRECTION ( 'NONE',  ( 0.000000000000000000, 0.000000000000000000, 1.000000000000000000 ) ) ;
#5177=ORIENTED_EDGE ( 'NONE', *, *, #3355, .F. ) ;
#5178=EDGE_LOOP ( 'NONE', ( #5334, #5273, #1814, #560 ) ) ;
#5180=CARTESIAN_POINT ( 'NONE',  ( 80.00000000000000000, 9.797174393178826052E-15, 40.00000000000000000 ) ) ;
#5182=FACE_OUTER_BOUND ( 'NONE', #5775, .T. ) ;
#5184=EDGE_CURVE ( 'NONE', #6052, #2828, #5208, .T. ) ;
#5186=ORIENTED_EDGE ( 'NONE', *, *, #1839, .F. ) ;
#5190=EDGE_LOOP ( 'NONE', ( #724, #4700, #4990, #4259 ) ) ;
#5191=CARTESIAN_POINT ( 'NONE',  ( 52.58482424179591419, -72.37680137756305498, -40.00000000000000000 ) ) ;
#5192=EDGE_CURVE ( 'NONE', #3886, #1883, #5528, .T. ) ;
#5196=ORIENTED_EDGE ( 'NONE', *, *, #5649, .F. ) ;
#5197=DIRECTION ( 'NONE',  ( 0.6273063437270329779, -0.7787725926866080339, 0.000000000000000000 ) ) ;
#5198=ORIENTED_EDGE ( 'NONE', *, *, #1511, .F. ) ;
#5199=CARTESIAN_POINT ( 'NONE',  ( 9.074396217167167933, 58.26942451214404173, 35.00000000000000000 ) ) ;
#5202=VERTEX_POINT ( 'NONE', #4737 ) ;
#5203=CARTESIAN_POINT ( 'NONE',  ( 9.192833548570416013, -59.02994620156847105, 35.00000000000000000 ) ) ;
#5207=DIRECTION ( 'NONE',  ( -0.000000000000000000, 0.000000000000000000, 1.000000000000000000 ) ) ;
#5208=LINE ( 'NONE', #1021, #2437 ) ;
#5211=EDGE_CURVE ( 'NONE', #413, #2151, #3395, .T. ) ;
#5213=ADVANCED_FACE ( 'NONE', ( #2074 ), #2927, .F. ) ;
#5214=PLANE ( 'NONE',  #1668 ) ;
#5217=ORIENTED_EDGE ( 'NONE', *, *, #4993, .T. ) ;
#5220=CYLINDRICAL_SURFACE ( 'NONE', #2737, 4.999999999999990230 ) ;
#5221=EDGE_CURVE ( 'NONE', #6071, #1883, #1626, .T. ) ;
#5222=ORIENTED_EDGE ( 'NONE', *, *, #5883, .F. ) ;
#5230=CARTESIAN_POINT ( 'NONE',  ( -100.0000000000000000, 0.000000000000000000, -39.00000000000002842 ) ) ;
#5231=AXIS2_PLACEMENT_3D ( 'NONE', #5656, #1380, #1783 ) ;
#5232=ORIENTED_EDGE ( 'NONE', *, *, #4300, .T. ) ;
#5233=DIRECTION ( 'NONE',  ( 1.000000000000000000, 0.000000000000000000, 0.000000000000000000 ) ) ;
#5234=AXIS2_PLACEMENT_3D ( 'NONE', #465, #2695, #5161 ) ;
#5236=VECTOR ( 'NONE', #4568, 1000.000000000000114 ) ;
#5237=DIRECTION ( 'NONE',  ( 1.000000000000000000, 0.000000000000000000, 0.000000000000000000 ) ) ;
#5243=VERTEX_POINT ( 'NONE', #592 ) ;
#5244=ORIENTED_EDGE ( 'NONE', *, *, #4466, .T. ) ;
#5245=DIRECTION ( 'NONE',  ( -0.000000000000000000, -0.000000000000000000, -1.000000000000000000 ) ) ;
#5246=DIRECTION ( 'NONE',  ( 0.7787725926866163606, -0.6273063437270225418, 0.000000000000000000 ) ) ;
#5247=DIRECTION ( 'NONE',  ( -0.000000000000000000, -0.000000000000000000, -1.000000000000000000 ) ) ;
#5249=CYLINDRICAL_SURFACE ( 'NONE', #4661, 80.00000000000000000 ) ;
#5250=FACE_OUTER_BOUND ( 'NONE', #3110, .T. ) ;
#5251=ORIENTED_EDGE ( 'NONE', *, *, #3679, .F. ) ;
#5252=CIRCLE ( 'NONE', #5946, 12.50000000000000000 ) ;
#5256=VERTEX_POINT ( 'NONE', #4325 ) ;
#5257=DIRECTION ( 'NONE',  ( 0.1538769332794358846, 0.9880900209011910240, 0.000000000000000000 ) ) ;
#5258=AXIS2_PLACEMENT_3D ( 'NONE', #2302, #3149, #2273 ) ;
#5263=CIRCLE ( 'NONE', #889, 5.000000000000004441 ) ;
#5264=VECTOR ( 'NONE', #4543, 1000.000000000000000 ) ;
#5265=DIRECTION ( 'NONE',  ( -0.000000000000000000, -0.000000000000000000, -1.000000000000000000 ) ) ;
#5266=EDGE_CURVE ( 'NONE', #2727, #5910, #462, .T. ) ;
#5268=VECTOR ( 'NONE', #3719, 999.9999999999998863 ) ;
#5270=CARTESIAN_POINT ( 'NONE',  ( 67.92475106770454829, -25.56373185532678960, 35.00000000000000000 ) ) ;
#5273=ORIENTED_EDGE ( 'NONE', *, *, #5073, .T. ) ;
#5274=DIRECTION ( 'NONE',  ( -0.000000000000000000, -0.000000000000000000, -1.000000000000000000 ) ) ;
#5276=ORIENTED_EDGE ( 'NONE', *, *, #1846, .T. ) ;
#5279=DIRECTION ( 'NONE',  ( 1.000000000000000000, 0.000000000000000000, 0.000000000000000000 ) ) ;
#5282=DIRECTION ( 'NONE',  ( -0.000000000000000000, 0.000000000000000000, 1.000000000000000000 ) ) ;
#5288=ORIENTED_EDGE ( 'NONE', *, *, #1913, .F. ) ;
#5293=CARTESIAN_POINT ( 'NONE',  ( 80.08403291566592941, 27.64547812922851833, -40.00000000000000000 ) ) ;
#5294=CARTESIAN_POINT ( 'NONE',  ( 55.48030965892933608, 45.89047003626479437, 35.00000000000000000 ) ) ;
#5295=ORIENTED_EDGE ( 'NONE', *, *, #3030, .F. ) ;
#5300=ADVANCED_FACE ( 'NONE', ( #5483 ), #4595, .F. ) ;
#5301=FACE_BOUND ( 'NONE', #4927, .T. ) ;
#5303=ORIENTED_EDGE ( 'NONE', *, *, #3247, .F. ) ;
#5305=CARTESIAN_POINT ( 'NONE',  ( 0.000000000000000000, 0.000000000000000000, 35.00000000000000000 ) ) ;
#5306=CARTESIAN_POINT ( 'NONE',  ( 5.114554293134526134E-14, 6.349488965209711204E-14, 35.00000000000000000 ) ) ;
#5307=LINE ( 'NONE', #1896, #4251 ) ;
#5309=EDGE_CURVE ( 'NONE', #4004, #1816, #2611, .T. ) ;
#5311=ORIENTED_EDGE ( 'NONE', *, *, #2710, .T. ) ;
#5314=DIRECTION ( 'NONE',  ( 0.000000000000000000, 0.000000000000000000, 1.000000000000000000 ) ) ;
#5316=DIRECTION ( 'NONE',  ( 0.000000000000000000, 0.000000000000000000, 1.000000000000000000 ) ) ;
#5320=CIRCLE ( 'NONE', #2923, 12.49999999999999822 ) ;
#5321=CARTESIAN_POINT ( 'NONE',  ( -62.30180741492890206, 50.18450749816231848, 35.00000000000000000 ) ) ;
#5322=DIRECTION ( 'NONE',  ( 0.000000000000000000, 0.000000000000000000, 1.000000000000000000 ) ) ;
#5323=EDGE_LOOP ( 'NONE', ( #828, #5122, #204, #985 ) ) ;
#5324=LINE ( 'NONE', #1074, #184 ) ;
#5326=AXIS2_PLACEMENT_3D ( 'NONE', #2169, #4062, #4118 ) ;
#5327=VECTOR ( 'NONE', #2207, 1000.000000000000114 ) ;
#5329=ORIENTED_EDGE ( 'NONE', *, *, #1788, .F. ) ;
#5332=CIRCLE ( 'NONE', #1935, 80.00000000000000000 ) ;
#5333=CIRCLE ( 'NONE', #2135, 80.00000000000000000 ) ;
#5334=ORIENTED_EDGE ( 'NONE', *, *, #698, .T. ) ;
#5336=ORIENTED_EDGE ( 'NONE', *, *, #5906, .T. ) ;
#5338=EDGE_CURVE ( 'NONE', #537, #730, #4501, .T. ) ;
#5339=DIRECTION ( 'NONE',  ( -0.9326495259660420034, -0.3607836771741717574, 0.000000000000000000 ) ) ;
#5341=AXIS2_PLACEMENT_3D ( 'NONE', #2282, #2347, #2252 ) ;
#5342=DIRECTION ( 'NONE',  ( -0.000000000000000000, -0.000000000000000000, -1.000000000000000000 ) ) ;
#5344=CONICAL_SURFACE ( 'NONE', #1943, 100.0000000000000000, 0.7853981633974621568 ) ;
#5345=VECTOR ( 'NONE', #5839, 1000.000000000000000 ) ;
#5346=VERTEX_POINT ( 'NONE', #5510 ) ;
#5347=EDGE_CURVE ( 'NONE', #5498, #1368, #2826, .T. ) ;
#5349=CARTESIAN_POINT ( 'NONE',  ( -57.35713647667095927, -46.20154318182582642, 35.13717928826310555 ) ) ;
#5350=VECTOR ( 'NONE', #4691, 1000.000000000000000 ) ;
#5351=ORIENTED_EDGE ( 'NONE', *, *, #1483, .T. ) ;
#5354=ORIENTED_EDGE ( 'NONE', *, *, #5826, .T. ) ;
#5355=FACE_OUTER_BOUND ( 'NONE', #1688, .T. ) ;
#5356=VECTOR ( 'NONE', #5247, 1000.000000000000000 ) ;
#5358=VECTOR ( 'NONE', #894, 1000.000000000000000 ) ;
#5359=CARTESIAN_POINT ( 'NONE',  ( 0.000000000000000000, 0.000000000000000000, 38.99999999999995737 ) ) ;
#5360=ORIENTED_EDGE ( 'NONE', *, *, #1669, .T. ) ;
#5362=AXIS2_PLACEMENT_3D ( 'NONE', #2493, #4380, #1546 ) ;
#5364=EDGE_CURVE ( 'NONE', #3660, #4090, #666, .T. ) ;
#5366=CARTESIAN_POINT ( 'NONE',  ( -45.92560378283280187, -36.99336990414421678, -35.00000000000000000 ) ) ;
#5367=AXIS2_PLACEMENT_3D ( 'NONE', #971, #3842, #4819 ) ;
#5369=VERTEX_POINT ( 'NONE', #1238 ) ;
#5370=VERTEX_POINT ( 'NONE', #5044 ) ;
#5374=CYLINDRICAL_SURFACE ( 'NONE', #4364, 12.49999999999999645 ) ;
#5375=CARTESIAN_POINT ( 'NONE',  ( 46.52501622030442974, -37.47620048660870395, 35.00000000000000000 ) ) ;
#5377=EDGE_CURVE ( 'NONE', #6119, #3856, #4029, .T. ) ;
#5380=DIRECTION ( 'NONE',  ( 1.000000000000000000, 0.000000000000000000, 0.000000000000000000 ) ) ;
#5382=CARTESIAN_POINT ( 'NONE',  ( 57.35713647667095927, 46.20154318182582642, 35.13717928826310555 ) ) ;
#5385=ADVANCED_FACE ( 'NONE', ( #4570 ), #4112, .F. ) ;
#5387=ORIENTED_EDGE ( 'NONE', *, *, #5309, .F. ) ;
#5392=DIRECTION ( 'NONE',  ( 1.000000000000000000, 0.000000000000000000, 0.000000000000000000 ) ) ;
#5393=DIRECTION ( 'NONE',  ( -0.000000000000000000, -0.000000000000000000, -1.000000000000000000 ) ) ;
#5397=EDGE_LOOP ( 'NONE', ( #2466, #2960, #110, #28 ) ) ;
#5398=CARTESIAN_POINT ( 'NONE',  ( 85.08403291566575888, -27.64547812922912939, 40.00000000000000000 ) ) ;
#5399=DIRECTION ( 'NONE',  ( 1.000000000000000000, 0.000000000000000000, 0.000000000000000000 ) ) ;
#5401=FACE_OUTER_BOUND ( 'NONE', #1429, .T. ) ;
#5403=EDGE_LOOP ( 'NONE', ( #5303, #4373, #2934, #1851, #2762, #2031 ) ) ;
#5406=( LENGTH_UNIT ( ) NAMED_UNIT ( * ) SI_UNIT ( .MILLI., .METRE. ) );
#5407=ADVANCED_FACE ( 'NONE', ( #2130 ), #227, .F. ) ;
#5409=ORIENTED_EDGE ( 'NONE', *, *, #2161, .T. ) ;
#5412=ORIENTED_EDGE ( 'NONE', *, *, #2518, .F. ) ;
#5413=FACE_BOUND ( 'NONE', #5081, .T. ) ;
#5414=ADVANCED_FACE ( 'NONE', ( #3622 ), #1267, .F. ) ;
#5416=DIRECTION ( 'NONE',  ( -0.6273063437270228748, -0.7787725926866162496, 0.000000000000000000 ) ) ;
#5417=EDGE_LOOP ( 'NONE', ( #2180, #5155, #5601, #4870 ) ) ;
#5418=LINE ( 'NONE', #2102, #4123 ) ;
#5419=EDGE_CURVE ( 'NONE', #6071, #6127, #4622, .T. ) ;
#5421=ORIENTED_EDGE ( 'NONE', *, *, #1322, .F. ) ;
#5422=CARTESIAN_POINT ( 'NONE',  ( 0.000000000000000000, 0.000000000000000000, 38.99999999999995737 ) ) ;
#5424=VERTEX_POINT ( 'NONE', #5571 ) ;
#5425=LINE ( 'NONE', #264, #5159 ) ;
#5426=CIRCLE ( 'NONE', #4936, 12.49999999999999822 ) ;
#5429=DIRECTION ( 'NONE',  ( 0.000000000000000000, 0.000000000000000000, 1.000000000000000000 ) ) ;
#5431=AXIS2_PLACEMENT_3D ( 'NONE', #2817, #2354, #4245 ) ;
#5433=ORIENTED_EDGE ( 'NONE', *, *, #2781, .T. ) ;
#5436=DIRECTION ( 'NONE',  ( 0.000000000000000000, 0.000000000000000000, 1.000000000000000000 ) ) ;
#5438=AXIS2_PLACEMENT_3D ( 'NONE', #4402, #507, #1877 ) ;
#5439=VECTOR ( 'NONE', #5622, 1000.000000000000000 ) ;
#5440=ORIENTED_EDGE ( 'NONE', *, *, #5471, .F. ) ;
#5441=ADVANCED_FACE ( 'NONE', ( #1296 ), #4982, .F. ) ;
#5442=LINE ( 'NONE', #3005, #5918 ) ;
#5444=VERTEX_POINT ( 'NONE', #4279 ) ;
#5445=AXIS2_PLACEMENT_3D ( 'NONE', #5509, #4116, #6091 ) ;
#5447=DIRECTION ( 'NONE',  ( -1.000000000000000000, 0.000000000000000000, 0.000000000000000000 ) ) ;
#5449=ADVANCED_FACE ( 'NONE', ( #4756 ), #510, .F. ) ;
#5451=AXIS2_PLACEMENT_3D ( 'NONE', #2964, #2471, #4362 ) ;
#5452=DIRECTION ( 'NONE',  ( 1.000000000000000000, 0.000000000000000000, 0.000000000000000000 ) ) ;
#5455=EDGE_CURVE ( 'NONE', #506, #6119, #4526, .T. ) ;
#5456=FACE_BOUND ( 'NONE', #4085, .T. ) ;
#5457=CIRCLE ( 'NONE', #3352, 12.50000000000138556 ) ;
#5462=AXIS2_PLACEMENT_3D ( 'NONE', #4164, #3694, #3207 ) ;
#5464=DIRECTION ( 'NONE',  ( -1.000000000000000000, 0.000000000000000000, 0.000000000000000000 ) ) ;
#5465=DIRECTION ( 'NONE',  ( -0.000000000000000000, -0.000000000000000000, -1.000000000000000000 ) ) ;
#5467=VECTOR ( 'NONE', #5108, 1000.000000000000227 ) ;
#5468=CARTESIAN_POINT ( 'NONE',  ( 58.45671475544921947, 33.75000000000068212, -35.00000000000000000 ) ) ;
#5470=CIRCLE ( 'NONE', #5367, 5.000000000000003553 ) ;
#5471=EDGE_CURVE ( 'NONE', #4471, #3966, #1341, .T. ) ;
#5472=ORIENTED_EDGE ( 'NONE', *, *, #208, .F. ) ;
#5476=ORIENTED_EDGE ( 'NONE', *, *, #5486, .T. ) ;
#5479=ORIENTED_EDGE ( 'NONE', *, *, #4495, .T. ) ;
#5481=LINE ( 'NONE', #5976, #573 ) ;
#5483=FACE_OUTER_BOUND ( 'NONE', #2624, .T. ) ;
#5486=EDGE_CURVE ( 'NONE', #3675, #1974, #3317, .T. ) ;
#5489=ORIENTED_EDGE ( 'NONE', *, *, #5841, .F. ) ;
#5491=VERTEX_POINT ( 'NONE', #5623 ) ;
#5493=CARTESIAN_POINT ( 'NONE',  ( 55.71784976887403928, 21.55374571496248137, -35.00000000000000000 ) ) ;
#5495=ADVANCED_FACE ( 'NONE', ( #6123 ), #4687, .F. ) ;
#5498=VERTEX_POINT ( 'NONE', #5661 ) ;
#5500=DIRECTION ( 'NONE',  ( 1.000000000000000000, 0.000000000000000000, 0.000000000000000000 ) ) ;
#5501=DIRECTION ( 'NONE',  ( -0.6273063437270329779, 0.7787725926866080339, 0.000000000000000000 ) ) ;
#5502=EDGE_CURVE ( 'NONE', #2370, #3250, #5332, .T. ) ;
#5503=VERTEX_POINT ( 'NONE', #470 ) ;
#5504=LINE ( 'NONE', #697, #258 ) ;
#5506=ORIENTED_EDGE ( 'NONE', *, *, #5377, .F. ) ;
#5507=FACE_BOUND ( 'NONE', #2498, .T. ) ;
#5509=CARTESIAN_POINT ( 'NONE',  ( 52.58482424179591419, -72.37680137756305498, -40.00000000000000000 ) ) ;
#5510=CARTESIAN_POINT ( 'NONE',  ( -9.074396217167167933, -58.26942451214404173, 35.00000000000000000 ) ) ;
#5513=ORIENTED_EDGE ( 'NONE', *, *, #48, .T. ) ;
#5518=CARTESIAN_POINT ( 'NONE',  ( -8.056095891487838412E-14, 1.254589464284425060E-14, 35.00000000000000000 ) ) ;
#5521=EDGE_CURVE ( 'NONE', #3966, #4001, #3221, .T. ) ;
#5522=EDGE_CURVE ( 'NONE', #1135, #3734, #3929, .T. ) ;
#5523=ORIENTED_EDGE ( 'NONE', *, *, #6011, .F. ) ;
#5525=CARTESIAN_POINT ( 'NONE',  ( -52.58482424179536707, 72.37680137756343868, -40.00000000000000000 ) ) ;
#5527=DIRECTION ( 'NONE',  ( -0.4999999999999919509, -0.8660254037844432595, 0.000000000000000000 ) ) ;
#5528=CIRCLE ( 'NONE', #1436, 10.00000000000000711 ) ;
#5529=AXIS2_PLACEMENT_3D ( 'NONE', #979, #3358, #5669 ) ;
#5532=EDGE_CURVE ( 'NONE', #3836, #4001, #411, .T. ) ;
#5537=CARTESIAN_POINT ( 'NONE',  ( 0.000000000000000000, 0.000000000000000000, 35.00000000000000000 ) ) ;
#5540=CIRCLE ( 'NONE', #4328, 12.50000000000138911 ) ;
#5541=CARTESIAN_POINT ( 'NONE',  ( -55.00000000000000711, -2.463307335887066074E-13, 35.00000000000000000 ) ) ;
#5542=DIRECTION ( 'NONE',  ( 0.3607836771741465554, 0.9326495259660518844, -0.000000000000000000 ) ) ;
#5546=ORIENTED_EDGE ( 'NONE', *, *, #2743, .T. ) ;
#5548=EDGE_LOOP ( 'NONE', ( #1503, #631 ) ) ;
#5549=CARTESIAN_POINT ( 'NONE',  ( 58.45671475544921947, 33.75000000000068212, 35.00000000000000000 ) ) ;
#5551=AXIS2_PLACEMENT_3D ( 'NONE', #1223, #4393, #5399 ) ;
#5552=DIRECTION ( 'NONE',  ( -0.000000000000000000, -0.000000000000000000, 1.000000000000000000 ) ) ;
#5554=LINE ( 'NONE', #3180, #2865 ) ;
#5555=AXIS2_PLACEMENT_3D ( 'NONE', #1765, #1220, #4160 ) ;
#5556=ORIENTED_EDGE ( 'NONE', *, *, #1788, .T. ) ;
#5557=CARTESIAN_POINT ( 'NONE',  ( -52.58482424179695158, -72.37680137756228760, -79.99999999999998579 ) ) ;
#5558=CARTESIAN_POINT ( 'NONE',  ( -57.58482424179695869, -72.37680137756228760, -40.00000000000000000 ) ) ;
#5560=EDGE_CURVE ( 'NONE', #5943, #2132, #5931, .T. ) ;
#5564=ORIENTED_EDGE ( 'NONE', *, *, #2629, .T. ) ;
#5566=CARTESIAN_POINT ( 'NONE',  ( 80.08403291566592941, 27.64547812922851833, 40.00000000000000000 ) ) ;
#5568=CARTESIAN_POINT ( 'NONE',  ( 5.114554293134526134E-14, 6.349488965209711204E-14, -35.00000000000000000 ) ) ;
#5570=LINE ( 'NONE', #5541, #5439 ) ;
#5571=CARTESIAN_POINT ( 'NONE',  ( 9.074396217167732814, -58.26942451214393515, 35.00000000000000000 ) ) ;
#5574=VERTEX_POINT ( 'NONE', #3875 ) ;
#5575=DIRECTION ( 'NONE',  ( 0.3607836771741465554, 0.9326495259660518844, -0.000000000000000000 ) ) ;
#5576=ORIENTED_EDGE ( 'NONE', *, *, #1129, .T. ) ;
#5577=DIRECTION ( 'NONE',  ( -0.000000000000000000, -0.000000000000000000, -1.000000000000000000 ) ) ;
#5578=CARTESIAN_POINT ( 'NONE',  ( 100.0000000000000000, 0.000000000000000000, -39.00000000000002842 ) ) ;
#5579=CARTESIAN_POINT ( 'NONE',  ( -62.30180741492871022, -50.18450749816254586, 38.99999999999995737 ) ) ;
#5581=DIRECTION ( 'NONE',  ( -0.7787725926866115866, 0.6273063437270286480, 0.000000000000000000 ) ) ;
#5583=CARTESIAN_POINT ( 'NONE',  ( -58.45671475544968843, 33.74999999999987210, 35.00000000000000000 ) ) ;
#5584=DIRECTION ( 'NONE',  ( -0.000000000000000000, -0.000000000000000000, 1.000000000000000000 ) ) ;
#5589=ORIENTED_EDGE ( 'NONE', *, *, #5347, .T. ) ;
#5591=CARTESIAN_POINT ( 'NONE',  ( -1.131281550719566266E-13, -1.761763928569765259E-14, -35.00000000000000000 ) ) ;
#5592=DIRECTION ( 'NONE',  ( 1.000000000000000000, 0.000000000000000000, 0.000000000000000000 ) ) ;
#5593=CARTESIAN_POINT ( 'NONE',  ( 45.92560378283317135, -36.99336990414376913, 35.00000000000000000 ) ) ;
#5594=ADVANCED_FACE ( 'NONE', ( #5790 ), #1543, .F. ) ;
#5595=CARTESIAN_POINT ( 'NONE',  ( -72.00000000000004263, 0.000000000000000000, 45.00000000000000711 ) ) ;
#5598=ADVANCED_FACE ( 'NONE', ( #5355 ), #5620, .T. ) ;
#5601=ORIENTED_EDGE ( 'NONE', *, *, #138, .F. ) ;
#5603=DIRECTION ( 'NONE',  ( -0.000000000000000000, 0.000000000000000000, 1.000000000000000000 ) ) ;
#5604=CARTESIAN_POINT ( 'NONE',  ( 11.33314185116896589, 72.77350886803867525, -35.00000000000000000 ) ) ;
#5606=CARTESIAN_POINT ( 'NONE',  ( 85.08403291566592941, 27.64547812922851833, -40.00000000000000000 ) ) ;
#5610=CARTESIAN_POINT ( 'NONE',  ( 7.182140071210238271E-14, -8.916303653273167033E-14, 35.00000000000000000 ) ) ;
#5615=DIRECTION ( 'NONE',  ( -1.000000000000000000, 0.000000000000000000, 0.000000000000000000 ) ) ;
#5616=AXIS2_PLACEMENT_3D ( 'NONE', #5989, #3603, #804 ) ;
#5617=EDGE_CURVE ( 'NONE', #1135, #5804, #3161, .T. ) ;
#5618=ORIENTED_EDGE ( 'NONE', *, *, #2208, .T. ) ;
#5619=FACE_OUTER_BOUND ( 'NONE', #1623, .T. ) ;
#5620=CONICAL_SURFACE ( 'NONE', #2939, 100.0000000000000000, 0.7853981633974621568 ) ;
#5622=DIRECTION ( 'NONE',  ( -4.496403249731883200E-15, 1.000000000000000000, 0.000000000000000000 ) ) ;
#5623=CARTESIAN_POINT ( 'NONE',  ( -45.92560378283290845, 36.99336990414408888, -35.00000000000000000 ) ) ;
#5625=ADVANCED_FACE ( 'NONE', ( #2694 ), #1602, .T. ) ;
#5626=EDGE_CURVE ( 'NONE', #5444, #1185, #1250, .T. ) ;
#5629=ORIENTED_EDGE ( 'NONE', *, *, #1972, .F. ) ;
#5632=CYLINDRICAL_SURFACE ( 'NONE', #1730, 5.000000000000004441 ) ;
#5634=CARTESIAN_POINT ( 'NONE',  ( 45.92560378283317135, -36.99336990414376913, 35.00000000000000000 ) ) ;
#5635=CYLINDRICAL_SURFACE ( 'NONE', #5529, 12.50000000000139266 ) ;
#5636=ORIENTED_EDGE ( 'NONE', *, *, #3455, .T. ) ;
#5641=ORIENTED_EDGE ( 'NONE', *, *, #4383, .F. ) ;
#5643=DIRECTION ( 'NONE',  ( 1.000000000000000000, 0.000000000000000000, 0.000000000000000000 ) ) ;
#5645=DIRECTION ( 'NONE',  ( 1.000000000000000000, 0.000000000000000000, 0.000000000000000000 ) ) ;
#5646=AXIS2_PLACEMENT_3D ( 'NONE', #4994, #626, #142 ) ;
#5649=EDGE_CURVE ( 'NONE', #1046, #429, #5481, .T. ) ;
#5651=AXIS2_PLACEMENT_3D ( 'NONE', #3908, #3242, #5090 ) ;
#5654=AXIS2_PLACEMENT_3D ( 'NONE', #4609, #421, #4582 ) ;
#5656=CARTESIAN_POINT ( 'NONE',  ( -5.114554293134481958E-14, -6.349488965209747807E-14, 35.00000000000000000 ) ) ;
#5658=ORIENTED_EDGE ( 'NONE', *, *, #4805, .T. ) ;
#5659=CARTESIAN_POINT ( 'NONE',  ( -47.58482424179695158, -72.37680137756228760, -40.00000000000000000 ) ) ;
#5661=CARTESIAN_POINT ( 'NONE',  ( -90.08403291566611415, -27.64547812922793923, -40.00000000000000000 ) ) ;
#5663=LINE ( 'NONE', #5762, #3852 ) ;
#5664=ORIENTED_EDGE ( 'NONE', *, *, #1155, .F. ) ;
#5665=DIRECTION ( 'NONE',  ( 0.000000000000000000, 0.000000000000000000, 1.000000000000000000 ) ) ;
#5667=ADVANCED_FACE ( 'NONE', ( #2195 ), #3072, .F. ) ;
#5668=LINE ( 'NONE', #580, #989 ) ;
#5669=DIRECTION ( 'NONE',  ( -1.000000000000000000, 0.000000000000000000, 0.000000000000000000 ) ) ;
#5670=ORIENTED_EDGE ( 'NONE', *, *, #5682, .F. ) ;
#5672=CARTESIAN_POINT ( 'NONE',  ( -74.61196207728390561, 28.86269417393235059, 38.99999999999995737 ) ) ;
#5673=EDGE_LOOP ( 'NONE', ( #4692, #4226 ) ) ;
#5674=ORIENTED_EDGE ( 'NONE', *, *, #334, .F. ) ;
#5675=DIRECTION ( 'NONE',  ( -0.000000000000000000, 0.000000000000000000, 1.000000000000000000 ) ) ;
#5680=FACE_OUTER_BOUND ( 'NONE', #1118, .T. ) ;
#5681=ORIENTED_EDGE ( 'NONE', *, *, #2978, .T. ) ;
#5682=EDGE_CURVE ( 'NONE', #1918, #4312, #160, .T. ) ;
#5684=ORIENTED_EDGE ( 'NONE', *, *, #6012, .T. ) ;
#5685=CARTESIAN_POINT ( 'NONE',  ( -55.00000000000000711, -2.463307335887066074E-13, 35.00000000000000000 ) ) ;
#5688=CARTESIAN_POINT ( 'NONE',  ( 12.00215801354989154, -70.99259259259225985, 35.00000000000000000 ) ) ;
#5695=DIRECTION ( 'NONE',  ( 0.000000000000000000, 0.000000000000000000, 1.000000000000000000 ) ) ;
#5697=DIRECTION ( 'NONE',  ( -0.000000000000000000, -0.000000000000000000, 1.000000000000000000 ) ) ;
#5701=ORIENTED_EDGE ( 'NONE', *, *, #2491, .T. ) ;
#5702=ORIENTED_EDGE ( 'NONE', *, *, #4138, .T. ) ;
#5704=LINE ( 'NONE', #3762, #5356 ) ;
#5707=DIRECTION ( 'NONE',  ( -0.000000000000000000, -0.000000000000000000, 1.000000000000000000 ) ) ;
#5708=EDGE_CURVE ( 'NONE', #6071, #5369, #5911, .T. ) ;
#5709=ADVANCED_FACE ( 'NONE', ( #2124 ), #4530, .F. ) ;
#5715=EDGE_CURVE ( 'NONE', #4988, #906, #1624, .T. ) ;
#5716=DIRECTION ( 'NONE',  ( 0.8660254037844385966, -0.5000000000000001110, 0.000000000000000000 ) ) ;
#5717=ADVANCED_FACE ( 'NONE', ( #5507, #3616, #3561, #4472, #3499, #1264, #5008, #5413, #3127, #753, #2634, #1151 ), #284, .F. ) ;
#5719=VECTOR ( 'NONE', #838, 1000.000000000000000 ) ;
#5720=DIRECTION ( 'NONE',  ( -0.000000000000000000, 0.000000000000000000, 1.000000000000000000 ) ) ;
#5722=AXIS2_PLACEMENT_3D ( 'NONE', #5595, #934, #1320 ) ;
#5723=CIRCLE ( 'NONE', #1153, 12.49999999999999822 ) ;
#5726=CIRCLE ( 'NONE', #5341, 72.00000000000004263 ) ;
#5728=DIRECTION ( 'NONE',  ( -0.000000000000000000, -0.000000000000000000, 1.000000000000000000 ) ) ;
#5729=CIRCLE ( 'NONE', #3038, 12.50000000000138556 ) ;
#5731=CARTESIAN_POINT ( 'NONE',  ( 4.999999999999380940, -89.46264649666795776, -79.99999999999998579 ) ) ;
#5732=EDGE_LOOP ( 'NONE', ( #2308, #4780, #1327, #1721 ) ) ;
#5733=DIRECTION ( 'NONE',  ( -0.000000000000000000, 0.000000000000000000, 1.000000000000000000 ) ) ;
#5734=( GEOMETRIC_REPRESENTATION_CONTEXT ( 3 ) GLOBAL_UNCERTAINTY_ASSIGNED_CONTEXT ( ( #1385 ) ) GLOBAL_UNIT_ASSIGNED_CONTEXT ( ( #5406, #691, #3064 ) ) REPRESENTATION_CONTEXT ( 'NONE', 'WORKASPACE' ) );
#5737=VERTEX_POINT ( 'NONE', #6001 ) ;
#5738=ADVANCED_FACE ( 'NONE', ( #1714 ), #6086, .F. ) ;
#5739=ORIENTED_EDGE ( 'NONE', *, *, #1694, .F. ) ;
#5745=DIRECTION ( 'NONE',  ( 0.9326495259660421144, 0.3607836771741718129, 0.000000000000000000 ) ) ;
#5751=ADVANCED_FACE ( 'NONE', ( #2785 ), #6063, .F. ) ;
#5753=CARTESIAN_POINT ( 'NONE',  ( 8.056095891487838412E-14, -1.254589464284425060E-14, 35.00000000000000000 ) ) ;
#5754=VECTOR ( 'NONE', #4217, 1000.000000000000000 ) ;
#5757=VECTOR ( 'NONE', #3176, 1000.000000000000000 ) ;
#5759=EDGE_CURVE ( 'NONE', #5893, #4711, #1733, .T. ) ;
#5760=CIRCLE ( 'NONE', #3070, 5.000000000000004441 ) ;
#5762=CARTESIAN_POINT ( 'NONE',  ( -2.941541598353333735E-14, 7.604078429494112756E-14, 35.00000000000000000 ) ) ;
#5766=EDGE_CURVE ( 'NONE', #2468, #5369, #6117, .T. ) ;
#5767=FACE_OUTER_BOUND ( 'NONE', #1409, .T. ) ;
#5768=DIRECTION ( 'NONE',  ( -0.000000000000000000, -0.000000000000000000, 1.000000000000000000 ) ) ;
#5769=ORIENTED_EDGE ( 'NONE', *, *, #4573, .F. ) ;
#5770=FACE_BOUND ( 'NONE', #2645, .T. ) ;
#5773=VERTEX_POINT ( 'NONE', #844 ) ;
#5775=EDGE_LOOP ( 'NONE', ( #126, #5244, #4435, #3104, #4562, #4902, #16 ) ) ;
#5776=CARTESIAN_POINT ( 'NONE',  ( 47.58482424179642578, 72.37680137756268550, 40.00000000000000000 ) ) ;
#5780=DIRECTION ( 'NONE',  ( -0.000000000000000000, -0.000000000000000000, -1.000000000000000000 ) ) ;
#5782=VERTEX_POINT ( 'NONE', #3677 ) ;
#5785=CARTESIAN_POINT ( 'NONE',  ( 0.000000000000000000, 0.000000000000000000, 38.99999999999995737 ) ) ;
#5789=ORIENTED_EDGE ( 'NONE', *, *, #4206, .F. ) ;
#5790=FACE_OUTER_BOUND ( 'NONE', #2516, .T. ) ;
#5791=EDGE_CURVE ( 'NONE', #1495, #4773, #2690, .T. ) ;
#5794=VERTEX_POINT ( 'NONE', #4618 ) ;
#5801=ADVANCED_FACE ( 'NONE', ( #3703 ), #5220, .F. ) ;
#5804=VERTEX_POINT ( 'NONE', #872 ) ;
#5805=CARTESIAN_POINT ( 'NONE',  ( 90.08403291566575888, -27.64547812922912939, -79.99999999999998579 ) ) ;
#5809=ORIENTED_EDGE ( 'NONE', *, *, #4597, .F. ) ;
#5811=DIRECTION ( 'NONE',  ( 0.4999999999999976685, 0.8660254037844400399, 0.000000000000000000 ) ) ;
#5814=DIRECTION ( 'NONE',  ( -0.9326495259660493309, 0.3607836771741531612, 0.000000000000000000 ) ) ;
#5816=ORIENTED_EDGE ( 'NONE', *, *, #742, .F. ) ;
#5820=AXIS2_PLACEMENT_3D ( 'NONE', #4971, #1566, #5380 ) ;
#5823=EDGE_LOOP ( 'NONE', ( #4921, #4542, #2106, #6089, #446 ) ) ;
#5824=DIRECTION ( 'NONE',  ( 1.000000000000000000, 0.000000000000000000, 0.000000000000000000 ) ) ;
#5826=EDGE_CURVE ( 'NONE', #1202, #1681, #431, .T. ) ;
#5827=AXIS2_PLACEMENT_3D ( 'NONE', #387, #2234, #2681 ) ;
#5828=EDGE_CURVE ( 'NONE', #1252, #3886, #563, .T. ) ;
#5830=DIRECTION ( 'NONE',  ( 1.000000000000000000, 0.000000000000000000, 0.000000000000000000 ) ) ;
#5833=AXIS2_PLACEMENT_3D ( 'NONE', #5537, #4592, #345 ) ;
#5837=CARTESIAN_POINT ( 'NONE',  ( -4.130675435985315210E-14, -1.067806758184287486E-13, 35.00000000000000000 ) ) ;
#5838=ADVANCED_FACE ( 'NONE', ( #4681 ), #3736, .F. ) ;
#5839=DIRECTION ( 'NONE',  ( -0.000000000000000000, -0.000000000000000000, -1.000000000000000000 ) ) ;
#5841=EDGE_CURVE ( 'NONE', #4037, #3906, #5726, .T. ) ;
#5842=VECTOR ( 'NONE', #375, 1000.000000000000227 ) ;
#5843=CARTESIAN_POINT ( 'NONE',  ( 11.33314185117008677, -72.77350886804093477, 35.00000000000000000 ) ) ;
#5844=CARTESIAN_POINT ( 'NONE',  ( -12.50000000000155254, 67.50000000000002842, 35.00000000000000000 ) ) ;
#5847=CARTESIAN_POINT ( 'NONE',  ( 27.50000000000000355, 47.63139720814412215, -35.00000000000000000 ) ) ;
#5849=CARTESIAN_POINT ( 'NONE',  ( 85.08403291566592941, 27.64547812922851833, -79.99999999999998579 ) ) ;
#5850=EDGE_CURVE ( 'NONE', #2489, #5243, #5098, .T. ) ;
#5851=VERTEX_POINT ( 'NONE', #5566 ) ;
#5852=DIRECTION ( 'NONE',  ( -1.000000000000000000, 0.000000000000000000, 0.000000000000000000 ) ) ;
#5854=VERTEX_POINT ( 'NONE', #4174 ) ;
#5856=CIRCLE ( 'NONE', #1090, 12.50000000000000355 ) ;
#5860=CARTESIAN_POINT ( 'NONE',  ( -67.48246767247867695, 25.10212255632726297, 35.00000000000000000 ) ) ;
#5861=ORIENTED_EDGE ( 'NONE', *, *, #5897, .F. ) ;
#5862=CARTESIAN_POINT ( 'NONE',  ( -52.58482424179695158, -72.37680137756228760, 40.00000000000000000 ) ) ;
#5863=VECTOR ( 'NONE', #807, 1000.000000000000000 ) ;
#5865=AXIS2_PLACEMENT_3D ( 'NONE', #2400, #3360, #1460 ) ;
#5867=ADVANCED_FACE ( 'NONE', ( #1412 ), #3238, .F. ) ;
#5870=ORIENTED_EDGE ( 'NONE', *, *, #2631, .T. ) ;
#5873=VECTOR ( 'NONE', #1898, 1000.000000000000000 ) ;
#5874=CARTESIAN_POINT ( 'NONE',  ( -45.92560378283290845, 36.99336990414408888, 35.00000000000000000 ) ) ;
#5876=EDGE_CURVE ( 'NONE', #1165, #5015, #3824, .T. ) ;
#5877=EDGE_LOOP ( 'NONE', ( #291, #6041, #4730, #5546 ) ) ;
#5879=CARTESIAN_POINT ( 'NONE',  ( -27.50000000000010303, 47.63139720814406530, 35.00000000000000000 ) ) ;
#5880=CARTESIAN_POINT ( 'NONE',  ( -90.08403291566611415, -27.64547812922793923, 40.00000000000000000 ) ) ;
#5881=VERTEX_POINT ( 'NONE', #4149 ) ;
#5883=EDGE_CURVE ( 'NONE', #2261, #1931, #3720, .T. ) ;
#5885=ORIENTED_EDGE ( 'NONE', *, *, #324, .T. ) ;
#5889=ORIENTED_EDGE ( 'NONE', *, *, #1333, .F. ) ;
#5890=CARTESIAN_POINT ( 'NONE',  ( -57.35713647666923976, 46.20154318182412112, 35.13717928826270054 ) ) ;
#5893=VERTEX_POINT ( 'NONE', #148 ) ;
#5897=EDGE_CURVE ( 'NONE', #1998, #5370, #2644, .T. ) ;
#5898=DIRECTION ( 'NONE',  ( 0.9326495259660420034, 0.3607836771741718129, 0.000000000000000000 ) ) ;
#5900=LINE ( 'NONE', #5874, #5075 ) ;
#5901=CARTESIAN_POINT ( 'NONE',  ( -85.08403291566554572, 27.64547812922971914, 40.00000000000000000 ) ) ;
#5902=EDGE_LOOP ( 'NONE', ( #869, #3869, #2718, #2292 ) ) ;
#5905=ADVANCED_FACE ( 'NONE', ( #27 ), #1058, .F. ) ;
#5906=EDGE_CURVE ( 'NONE', #4527, #1495, #4222, .T. ) ;
#5907=ORIENTED_EDGE ( 'NONE', *, *, #1442, .T. ) ;
#5910=VERTEX_POINT ( 'NONE', #4337 ) ;
#5911=LINE ( 'NONE', #4057, #1723 ) ;
#5912=ADVANCED_FACE ( 'NONE', ( #2029 ), #4912, .F. ) ;
#5913=EDGE_CURVE ( 'NONE', #3470, #4790, #1547, .T. ) ;
#5915=CARTESIAN_POINT ( 'NONE',  ( 0.000000000000000000, 0.000000000000000000, 45.00000000000000711 ) ) ;
#5916=VERTEX_POINT ( 'NONE', #5382 ) ;
#5918=VECTOR ( 'NONE', #1176, 1000.000000000000000 ) ;
#5919=CARTESIAN_POINT ( 'NONE',  ( 27.50000000000043698, -47.63139720814386635, -35.00000000000000000 ) ) ;
#5921=ORIENTED_EDGE ( 'NONE', *, *, #1736, .T. ) ;
#5923=AXIS2_PLACEMENT_3D ( 'NONE', #4951, #3366, #554 ) ;
#5924=ORIENTED_EDGE ( 'NONE', *, *, #6088, .F. ) ;
#5926=VECTOR ( 'NONE', #2557, 1000.000000000000000 ) ;
#5927=DIRECTION ( 'NONE',  ( -0.5000000000000042188, 0.8660254037844362651, 0.000000000000000000 ) ) ;
#5930=DIRECTION ( 'NONE',  ( 1.000000000000000000, 0.000000000000000000, 0.000000000000000000 ) ) ;
#5931=CIRCLE ( 'NONE', #5431, 80.00000000000002842 ) ;
#5933=VECTOR ( 'NONE', #2253, 1000.000000000000000 ) ;
#5934=ORIENTED_EDGE ( 'NONE', *, *, #1318, .F. ) ;
#5935=CYLINDRICAL_SURFACE ( 'NONE', #1535, 5.000000000000004441 ) ;
#5937=LINE ( 'NONE', #4974, #3137 ) ;
#5938=AXIS2_PLACEMENT_3D ( 'NONE', #645, #4382, #2012 ) ;
#5939=ORIENTED_EDGE ( 'NONE', *, *, #4249, .F. ) ;
#5940=PLANE ( 'NONE',  #277 ) ;
#5943=VERTEX_POINT ( 'NONE', #4276 ) ;
#5945=DIRECTION ( 'NONE',  ( -0.000000000000000000, -0.000000000000000000, 1.000000000000000000 ) ) ;
#5946=AXIS2_PLACEMENT_3D ( 'NONE', #1970, #3867, #5811 ) ;
#5948=EDGE_CURVE ( 'NONE', #2604, #836, #1637, .T. ) ;
#5949=CARTESIAN_POINT ( 'NONE',  ( 1.131281550719567528E-13, 1.761763928569687004E-14, -35.00000000000000000 ) ) ;
#5950=ORIENTED_EDGE ( 'NONE', *, *, #2427, .F. ) ;
#5952=CIRCLE ( 'NONE', #794, 5.000000000000004441 ) ;
#5954=EDGE_CURVE ( 'NONE', #2204, #4527, #1000, .T. ) ;
#5955=EDGE_LOOP ( 'NONE', ( #1377, #5409, #2909, #6129, #6097, #5513, #3313, #5641, #4012 ) ) ;
#5957=CIRCLE ( 'NONE', #5362, 9.999999999999996447 ) ;
#5958=EDGE_LOOP ( 'NONE', ( #1514, #5336, #1443, #5980, #3268, #3375, #734 ) ) ;
#5959=CARTESIAN_POINT ( 'NONE',  ( 11.82353433160560385, -71.60642589802972680, 35.00000000000000000 ) ) ;
#5960=LINE ( 'NONE', #4423, #2570 ) ;
#5961=CIRCLE ( 'NONE', #2760, 5.000000000000003553 ) ;
#5964=AXIS2_PLACEMENT_3D ( 'NONE', #741, #1142, #1679 ) ;
#5967=CIRCLE ( 'NONE', #511, 9.999999999999992895 ) ;
#5969=DIRECTION ( 'NONE',  ( 0.5000000000000103251, -0.8660254037844326014, 0.000000000000000000 ) ) ;
#5970=ORIENTED_EDGE ( 'NONE', *, *, #777, .F. ) ;
#5974=EDGE_LOOP ( 'NONE', ( #980, #3091, #902, #602 ) ) ;
#5976=CARTESIAN_POINT ( 'NONE',  ( -5.000000000000003553, 89.46264649666795776, -79.99999999999998579 ) ) ;
#5977=CARTESIAN_POINT ( 'NONE',  ( -80.08403291566554572, 27.64547812922971914, 40.00000000000000000 ) ) ;
#5979=CARTESIAN_POINT ( 'NONE',  ( -5.114554293134481958E-14, -6.349488965209747807E-14, -35.00000000000000000 ) ) ;
#5980=ORIENTED_EDGE ( 'NONE', *, *, #698, .F. ) ;
#5986=ORIENTED_EDGE ( 'NONE', *, *, #5791, .F. ) ;
#5987=DIRECTION ( 'NONE',  ( 0.5000000000000081046, -0.8660254037844340447, 0.000000000000000000 ) ) ;
#5988=DIRECTION ( 'NONE',  ( -1.000000000000000000, 0.000000000000000000, 0.000000000000000000 ) ) ;
#5989=CARTESIAN_POINT ( 'NONE',  ( 5.114554293134526134E-14, 6.349488965209711204E-14, 35.00000000000000000 ) ) ;
#5995=FACE_OUTER_BOUND ( 'NONE', #4864, .T. ) ;
#5996=VERTEX_POINT ( 'NONE', #2976 ) ;
#6001=CARTESIAN_POINT ( 'NONE',  ( 68.69027832783777399, 26.57196568621521138, -35.00000000000000000 ) ) ;
#6007=ORIENTED_EDGE ( 'NONE', *, *, #5826, .F. ) ;
#6008=DIRECTION ( 'NONE',  ( 0.000000000000000000, -0.000000000000000000, -1.000000000000000000 ) ) ;
#6010=DIRECTION ( 'NONE',  ( 0.8660254037844339337, 0.5000000000000079936, 0.000000000000000000 ) ) ;
#6011=EDGE_CURVE ( 'NONE', #2727, #1135, #3334, .T. ) ;
#6012=EDGE_CURVE ( 'NONE', #3856, #2123, #677, .T. ) ;
#6015=CARTESIAN_POINT ( 'NONE',  ( 0.000000000000000000, 0.000000000000000000, -40.00000000000000000 ) ) ;
#6017=DIRECTION ( 'NONE',  ( 1.000000000000000000, 0.000000000000000000, 0.000000000000000000 ) ) ;
#6018=AXIS2_PLACEMENT_3D ( 'NONE', #3537, #4534, #704 ) ;
#6020=DIRECTION ( 'NONE',  ( 0.3607836771741465554, 0.9326495259660518844, -0.000000000000000000 ) ) ;
#6021=EDGE_CURVE ( 'NONE', #5794, #670, #2943, .T. ) ;
#6023=CARTESIAN_POINT ( 'NONE',  ( -9.074396217167327805, 58.26942451214400620, 35.00000000000000000 ) ) ;
#6024=AXIS2_PLACEMENT_3D ( 'NONE', #3589, #3035, #699 ) ;
#6027=AXIS2_PLACEMENT_3D ( 'NONE', #4725, #5695, #3715 ) ;
#6033=DIRECTION ( 'NONE',  ( 1.000000000000000000, 0.000000000000000000, 0.000000000000000000 ) ) ;
#6035=DIRECTION ( 'NONE',  ( -0.9880900209011910240, 0.1538769332794358846, 0.000000000000000000 ) ) ;
#6036=DIRECTION ( 'NONE',  ( -0.000000000000000000, -0.000000000000000000, -1.000000000000000000 ) ) ;
#6038=DIRECTION ( 'NONE',  ( 0.9880900209011891366, 0.1538769332794488465, -0.000000000000000000 ) ) ;
#6039=DIRECTION ( 'NONE',  ( -1.000000000000000000, 0.000000000000000000, 0.000000000000000000 ) ) ;
#6040=VECTOR ( 'NONE', #3927, 1000.000000000000000 ) ;
#6041=ORIENTED_EDGE ( 'NONE', *, *, #2439, .F. ) ;
#6042=DIRECTION ( 'NONE',  ( 1.000000000000000000, 0.000000000000000000, 0.000000000000000000 ) ) ;
#6044=DIRECTION ( 'NONE',  ( 0.000000000000000000, 0.000000000000000000, 1.000000000000000000 ) ) ;
#6045=CARTESIAN_POINT ( 'NONE',  ( 62.30180741492871022, 50.18450749816254586, -35.00000000000000000 ) ) ;
#6052=VERTEX_POINT ( 'NONE', #4080 ) ;
#6055=DIRECTION ( 'NONE',  ( -0.3607836771741652626, 0.9326495259660447790, 0.000000000000000000 ) ) ;
#6058=ADVANCED_FACE ( 'NONE', ( #4492 ), #245, .F. ) ;
#6060=CIRCLE ( 'NONE', #4155, 5.000000000000003553 ) ;
#6063=PLANE ( 'NONE',  #5231 ) ;
#6064=DIRECTION ( 'NONE',  ( 0.000000000000000000, 0.000000000000000000, 1.000000000000000000 ) ) ;
#6066=DIRECTION ( 'NONE',  ( -0.000000000000000000, -0.000000000000000000, -1.000000000000000000 ) ) ;
#6067=DIRECTION ( 'NONE',  ( -0.000000000000000000, -0.000000000000000000, -1.000000000000000000 ) ) ;
#6069=ORIENTED_EDGE ( 'NONE', *, *, #392, .T. ) ;
#6070=PLANE ( 'NONE',  #1471 ) ;
#6071=VERTEX_POINT ( 'NONE', #1256 ) ;
#6073=CARTESIAN_POINT ( 'NONE',  ( -9.192833548570002122, 59.02994620156853500, -35.00000000000000000 ) ) ;
#6074=CARTESIAN_POINT ( 'NONE',  ( 0.000000000000000000, 0.000000000000000000, -35.00000000000000000 ) ) ;
#6077=EDGE_CURVE ( 'NONE', #5369, #4004, #868, .T. ) ;
#6079=CYLINDRICAL_SURFACE ( 'NONE', #4244, 5.000000000000004441 ) ;
#6084=VERTEX_POINT ( 'NONE', #275 ) ;
#6086=CYLINDRICAL_SURFACE ( 'NONE', #371, 80.00000000000000000 ) ;
#6087=ADVANCED_FACE ( 'NONE', ( #5995 ), #3094, .F. ) ;
#6088=EDGE_CURVE ( 'NONE', #4900, #3566, #5937, .T. ) ;
#6089=ORIENTED_EDGE ( 'NONE', *, *, #1662, .T. ) ;
#6091=DIRECTION ( 'NONE',  ( 1.000000000000000000, 0.000000000000000000, 0.000000000000000000 ) ) ;
#6096=LINE ( 'NONE', #2203, #2368 ) ;
#6097=ORIENTED_EDGE ( 'NONE', *, *, #2631, .F. ) ;
#6098=FACE_OUTER_BOUND ( 'NONE', #4745, .T. ) ;
#6099=ADVANCED_FACE ( 'NONE', ( #188 ), #4047, .F. ) ;
#6100=DIRECTION ( 'NONE',  ( -0.000000000000000000, -0.000000000000000000, -1.000000000000000000 ) ) ;
#6106=ORIENTED_EDGE ( 'NONE', *, *, #21, .F. ) ;
#6108=CARTESIAN_POINT ( 'NONE',  ( -12.31015466235523981, 79.04720167209522685, 35.00000000000000000 ) ) ;
#6109=CARTESIAN_POINT ( 'NONE',  ( -67.15076586955525784, -25.97642475653991312, 45.00000000000000711 ) ) ;
#6116=ORIENTED_EDGE ( 'NONE', *, *, #818, .T. ) ;
#6117=LINE ( 'NONE', #5591, #5842 ) ;
#6118=CONICAL_SURFACE ( 'NONE', #2725, 80.99999999999998579, 0.7853981633974482790 ) ;
#6119=VERTEX_POINT ( 'NONE', #4554 ) ;
#6120=DIRECTION ( 'NONE',  ( 0.5000000000000099920, -0.8660254037844328234, 0.000000000000000000 ) ) ;
#6121=VECTOR ( 'NONE', #1353, 1000.000000000000000 ) ;
#6122=EDGE_CURVE ( 'NONE', #3175, #3262, #5540, .T. ) ;
#6123=FACE_OUTER_BOUND ( 'NONE', #947, .T. ) ;
#6124=AXIS2_PLACEMENT_3D ( 'NONE', #5849, #89, #3002 ) ;
#6125=EDGE_CURVE ( 'NONE', #2223, #5916, #3627, .T. ) ;
#6127=VERTEX_POINT ( 'NONE', #3965 ) ;
#6129=ORIENTED_EDGE ( 'NONE', *, *, #3841, .F. ) ;
#6133=DIRECTION ( 'NONE',  ( 0.7071067811865474617, 0.000000000000000000, 0.7071067811865474617 ) ) ;
#6135=FACE_BOUND ( 'NONE', #5548, .T. ) ;
#6138=ORIENTED_EDGE ( 'NONE', *, *, #848, .F. ) ;
#6139=ORIENTED_EDGE ( 'NONE', *, *, #5759, .T. ) ;
#6192=COLOUR_RGB('Off White',0.89,0.88,0.83);
#6193=FILL_AREA_STYLE_COLOUR('',#6192);
#6194=FILL_AREA_STYLE('',(#6193));
#6195=SURFACE_STYLE_FILL_AREA(#6194);
#6196=SURFACE_SIDE_STYLE('',(#6195));
#6197=SURFACE_STYLE_USAGE(.BOTH.,#6196);
#6198=PRESENTATION_STYLE_ASSIGNMENT((#6197));
ENDSEC;
END-ISO-10303-21;
